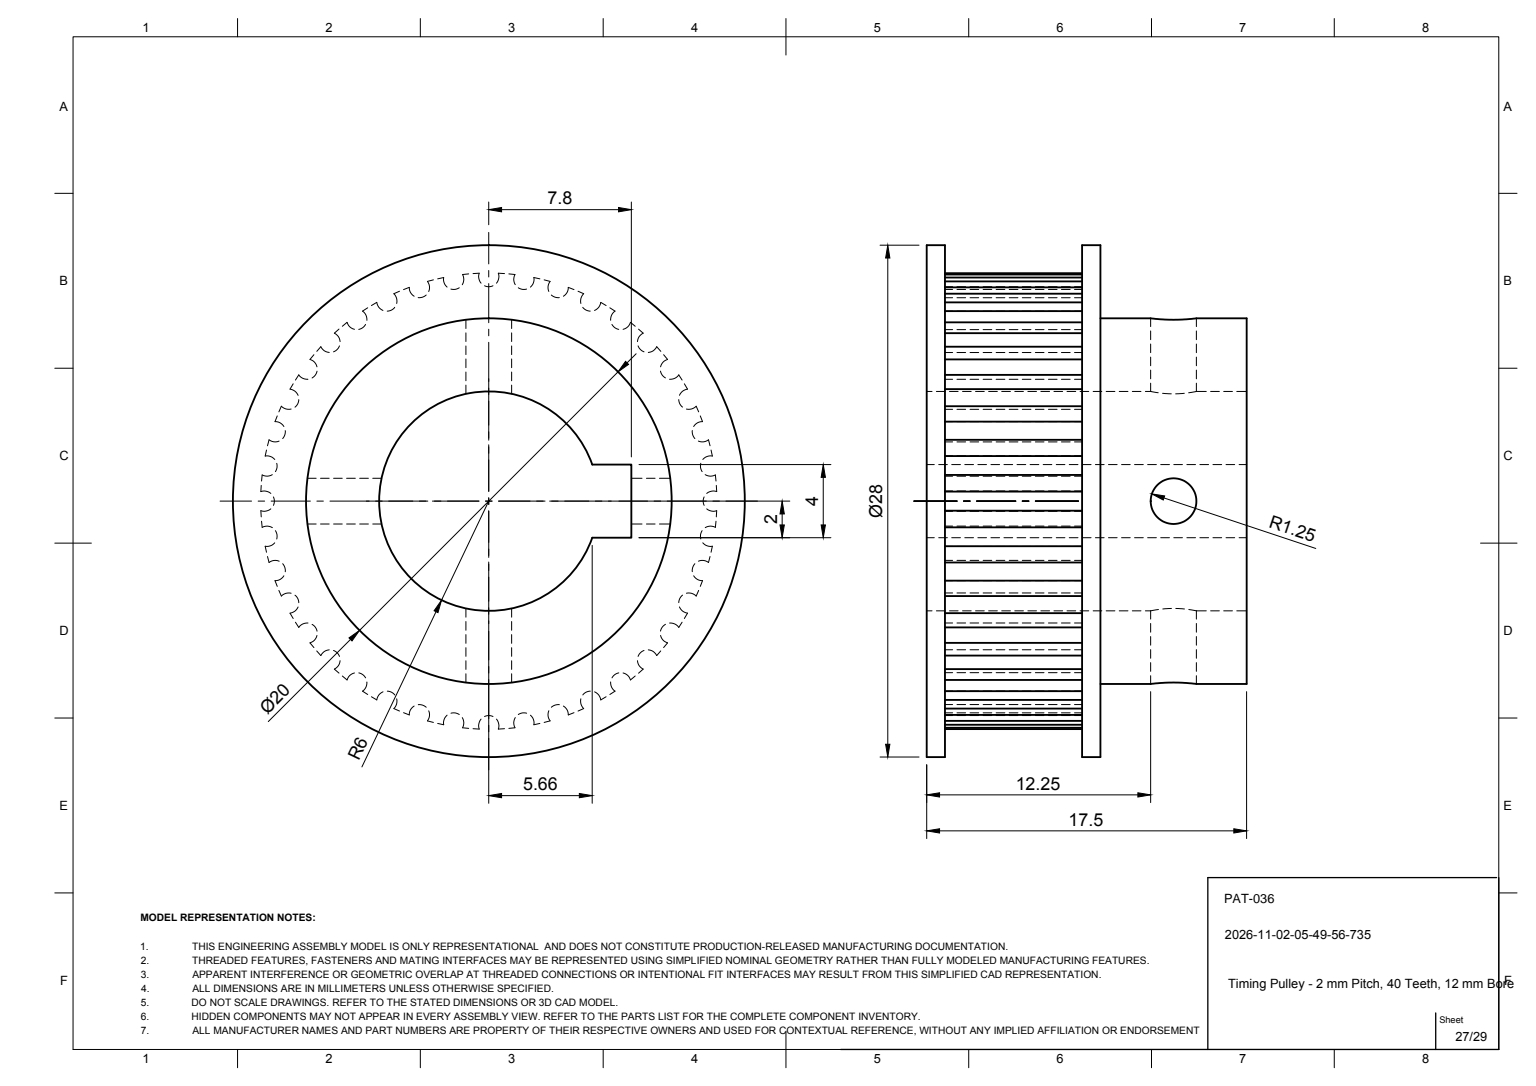
ISO-10303-21;
HEADER;
/* Generated by software containing ST-Developer
 * from STEP Tools, Inc. (www.steptools.com) 
 */

FILE_DESCRIPTION(
/* description */ ('Flange-mounted spindle'),
/* implementation_level */ '2;1');

FILE_NAME(
/* name */ 'Timing Pulley - 2 mm Pitch, 40 Teeth, 12 mm Bore.step',
/* time_stamp */ '2026-10-27T10:49:51-07:00',
/* author */ (''),
/* organization */ (''),
/* preprocessor_version */ 'ST-DEVELOPER v20.2',
/* originating_system */ 'Autodesk Translation Framework v15.17.0.0',
/* authorisation */ '');

FILE_SCHEMA (('AUTOMOTIVE_DESIGN { 1 0 10303 214 3 1 1 }'));
ENDSEC;

DATA;
#10=MECHANICAL_DESIGN_GEOMETRIC_PRESENTATION_REPRESENTATION('',(#359),#11764);
#243=B_SPLINE_CURVE_WITH_KNOTS('',3,(#10553,#10554,#10555,#10556,#10557,
#10558,#10559,#10560,#10561,#10562,#10563,#10564,#10565,#10566,#10567,#10568,
#10569,#10570),.UNSPECIFIED.,.F.,.F.,(4,2,2,2,2,2,2,2,4),(0.,0.0472365751919841,
0.0944731503839683,0.14170659898184,0.188940047579712,0.236173496177583,
0.283406944775455,0.330643519967439,0.377880095159423),.UNSPECIFIED.);
#244=B_SPLINE_CURVE_WITH_KNOTS('',3,(#10571,#10572,#10573,#10574,#10575,
#10576,#10577,#10578,#10579,#10580,#10581,#10582,#10583,#10584,#10585,#10586,
#10587,#10588),.UNSPECIFIED.,.F.,.F.,(4,2,2,2,2,2,2,2,4),(0.377880095159423,
0.425116670351408,0.472353245543392,0.519586694141263,0.566820142739135,
0.614053591337007,0.661287039934879,0.708523615126863,0.755760190318847),
 .UNSPECIFIED.);
#245=B_SPLINE_CURVE_WITH_KNOTS('',3,(#10591,#10592,#10593,#10594,#10595,
#10596,#10597,#10598,#10599,#10600,#10601,#10602,#10603,#10604,#10605,#10606,
#10607,#10608),.UNSPECIFIED.,.F.,.F.,(4,2,2,2,2,2,2,2,4),(0.,0.0472365751919841,
0.0944731503839682,0.14170659898184,0.188940047579712,0.236173496177583,
0.283406944775455,0.330643519967439,0.377880095159423),.UNSPECIFIED.);
#246=B_SPLINE_CURVE_WITH_KNOTS('',3,(#10609,#10610,#10611,#10612,#10613,
#10614,#10615,#10616,#10617,#10618,#10619,#10620,#10621,#10622,#10623,#10624,
#10625,#10626),.UNSPECIFIED.,.F.,.F.,(4,2,2,2,2,2,2,2,4),(0.377880095159423,
0.425116670351408,0.472353245543392,0.519586694141263,0.566820142739135,
0.614053591337007,0.661287039934879,0.708523615126863,0.755760190318847),
 .UNSPECIFIED.);
#247=B_SPLINE_CURVE_WITH_KNOTS('',3,(#10629,#10630,#10631,#10632,#10633,
#10634,#10635,#10636,#10637,#10638,#10639,#10640,#10641,#10642,#10643,#10644,
#10645,#10646),.UNSPECIFIED.,.F.,.F.,(4,2,2,2,2,2,2,2,4),(0.,0.0472365751919841,
0.0944731503839683,0.14170659898184,0.188940047579712,0.236173496177583,
0.283406944775455,0.330643519967439,0.377880095159423),.UNSPECIFIED.);
#248=B_SPLINE_CURVE_WITH_KNOTS('',3,(#10647,#10648,#10649,#10650,#10651,
#10652,#10653,#10654,#10655,#10656,#10657,#10658,#10659,#10660,#10661,#10662,
#10663,#10664),.UNSPECIFIED.,.F.,.F.,(4,2,2,2,2,2,2,2,4),(0.377880095159423,
0.425116670351408,0.472353245543392,0.519586694141263,0.566820142739135,
0.614053591337007,0.661287039934879,0.708523615126863,0.755760190318847),
 .UNSPECIFIED.);
#249=B_SPLINE_CURVE_WITH_KNOTS('',3,(#10668,#10669,#10670,#10671,#10672,
#10673,#10674,#10675,#10676,#10677),.UNSPECIFIED.,.F.,.F.,(4,2,2,2,4),(0.565665723963061,
0.61280433739166,0.659942950820258,0.70708195805217,0.754220965284082),
 .UNSPECIFIED.);
#250=B_SPLINE_CURVE_WITH_KNOTS('',3,(#10679,#10680,#10681,#10682,#10683,
#10684,#10685,#10686,#10687,#10688,#10689,#10690,#10691,#10692,#10693,#10694,
#10695,#10696),.UNSPECIFIED.,.F.,.F.,(4,2,2,2,2,2,2,2,4),(0.18855524132102,
0.235693854749619,0.282832468178217,0.329971475410129,0.377110482642041,
0.424249489873953,0.471388497105864,0.518527110534463,0.565665723963061),
 .UNSPECIFIED.);
#251=B_SPLINE_CURVE_WITH_KNOTS('',3,(#10697,#10698,#10699,#10700,#10701,
#10702,#10703,#10704,#10705,#10706),.UNSPECIFIED.,.F.,.F.,(4,2,2,2,4),(0.754220965284082,
0.801359972515993,0.848498979747905,0.895637593176504,0.942776206605102),
 .UNSPECIFIED.);
#252=B_SPLINE_CURVE_WITH_KNOTS('',3,(#10712,#10713,#10714,#10715,#10716,
#10717,#10718,#10719,#10720,#10721),.UNSPECIFIED.,.F.,.F.,(4,2,2,2,4),(0.565665723963061,
0.61280433739166,0.659942950820258,0.70708195805217,0.754220965284082),
 .UNSPECIFIED.);
#253=B_SPLINE_CURVE_WITH_KNOTS('',3,(#10723,#10724,#10725,#10726,#10727,
#10728,#10729,#10730,#10731,#10732,#10733,#10734,#10735,#10736,#10737,#10738,
#10739,#10740),.UNSPECIFIED.,.F.,.F.,(4,2,2,2,2,2,2,2,4),(0.18855524132102,
0.235693854749619,0.282832468178217,0.329971475410129,0.377110482642041,
0.424249489873953,0.471388497105864,0.518527110534463,0.565665723963061),
 .UNSPECIFIED.);
#254=B_SPLINE_CURVE_WITH_KNOTS('',3,(#10741,#10742,#10743,#10744,#10745,
#10746,#10747,#10748,#10749,#10750),.UNSPECIFIED.,.F.,.F.,(4,2,2,2,4),(0.754220965284082,
0.801359972515993,0.848498979747905,0.895637593176504,0.942776206605102),
 .UNSPECIFIED.);
#255=B_SPLINE_CURVE_WITH_KNOTS('',3,(#10760,#10761,#10762,#10763,#10764,
#10765,#10766,#10767,#10768,#10769,#10770,#10771,#10772,#10773,#10774,#10775,
#10776,#10777),.UNSPECIFIED.,.F.,.F.,(4,2,2,2,2,2,2,2,4),(0.18855524132102,
0.235693854749619,0.282832468178217,0.329971475410129,0.377110482642041,
0.424249489873953,0.471388497105864,0.518527110534463,0.565665723963061),
 .UNSPECIFIED.);
#256=B_SPLINE_CURVE_WITH_KNOTS('',3,(#10779,#10780,#10781,#10782,#10783,
#10784,#10785,#10786,#10787,#10788),.UNSPECIFIED.,.F.,.F.,(4,2,2,2,4),(0.565665723963061,
0.61280433739166,0.659942950820258,0.70708195805217,0.754220965284082),
 .UNSPECIFIED.);
#257=B_SPLINE_CURVE_WITH_KNOTS('',3,(#10789,#10790,#10791,#10792,#10793,
#10794,#10795,#10796,#10797,#10798),.UNSPECIFIED.,.F.,.F.,(4,2,2,2,4),(0.754220965284082,
0.801359972515993,0.848498979747905,0.895637593176504,0.942776206605102),
 .UNSPECIFIED.);
#258=B_SPLINE_CURVE_WITH_KNOTS('',3,(#10801,#10802,#10803,#10804,#10805,
#10806,#10807,#10808,#10809,#10810,#10811,#10812,#10813,#10814,#10815,#10816,
#10817,#10818),.UNSPECIFIED.,.F.,.F.,(4,2,2,2,2,2,2,2,4),(0.18855524132102,
0.235693854749619,0.282832468178217,0.329971475410129,0.377110482642041,
0.424249489873953,0.471388497105864,0.518527110534463,0.565665723963061),
 .UNSPECIFIED.);
#259=B_SPLINE_CURVE_WITH_KNOTS('',3,(#10820,#10821,#10822,#10823,#10824,
#10825,#10826,#10827,#10828,#10829),.UNSPECIFIED.,.F.,.F.,(4,2,2,2,4),(0.565665723963061,
0.61280433739166,0.659942950820258,0.70708195805217,0.754220965284082),
 .UNSPECIFIED.);
#260=B_SPLINE_CURVE_WITH_KNOTS('',3,(#10830,#10831,#10832,#10833,#10834,
#10835,#10836,#10837,#10838,#10839),.UNSPECIFIED.,.F.,.F.,(4,2,2,2,4),(0.754220965284082,
0.801359972515993,0.848498979747905,0.895637593176504,0.942776206605102),
 .UNSPECIFIED.);
#304=SHAPE_REPRESENTATION_RELATIONSHIP('SRR','None',#11902,#331);
#331=ADVANCED_BREP_SHAPE_REPRESENTATION('',(#385),#11757);
#359=STYLED_ITEM('',(#12092),#385);
#385=MANIFOLD_SOLID_BREP('Body1',#6153);
#488=FACE_BOUND('',#1303,.T.);
#489=FACE_BOUND('',#1306,.T.);
#490=FACE_BOUND('',#1308,.T.);
#491=FACE_BOUND('',#1309,.T.);
#492=FACE_BOUND('',#1310,.T.);
#493=FACE_BOUND('',#1314,.T.);
#494=FACE_BOUND('',#1315,.T.);
#495=FACE_BOUND('',#1316,.T.);
#496=FACE_BOUND('',#1320,.T.);
#497=FACE_BOUND('',#1322,.T.);
#498=FACE_BOUND('',#1325,.T.);
#499=FACE_BOUND('',#1327,.T.);
#616=PLANE('',#6808);
#617=PLANE('',#6809);
#618=PLANE('',#6811);
#619=PLANE('',#6812);
#620=PLANE('',#6824);
#621=PLANE('',#6825);
#622=PLANE('',#6909);
#623=PLANE('',#6910);
#859=FACE_OUTER_BOUND('',#1301,.T.);
#860=FACE_OUTER_BOUND('',#1302,.T.);
#861=FACE_OUTER_BOUND('',#1304,.T.);
#862=FACE_OUTER_BOUND('',#1305,.T.);
#863=FACE_OUTER_BOUND('',#1307,.T.);
#864=FACE_OUTER_BOUND('',#1311,.T.);
#865=FACE_OUTER_BOUND('',#1312,.T.);
#866=FACE_OUTER_BOUND('',#1313,.T.);
#867=FACE_OUTER_BOUND('',#1317,.T.);
#868=FACE_OUTER_BOUND('',#1318,.T.);
#869=FACE_OUTER_BOUND('',#1319,.T.);
#870=FACE_OUTER_BOUND('',#1321,.T.);
#871=FACE_OUTER_BOUND('',#1323,.T.);
#872=FACE_OUTER_BOUND('',#1324,.T.);
#873=FACE_OUTER_BOUND('',#1326,.T.);
#874=FACE_OUTER_BOUND('',#1328,.T.);
#875=FACE_OUTER_BOUND('',#1329,.T.);
#876=FACE_OUTER_BOUND('',#1330,.T.);
#877=FACE_OUTER_BOUND('',#1331,.T.);
#878=FACE_OUTER_BOUND('',#1332,.T.);
#879=FACE_OUTER_BOUND('',#1333,.T.);
#880=FACE_OUTER_BOUND('',#1334,.T.);
#881=FACE_OUTER_BOUND('',#1335,.T.);
#882=FACE_OUTER_BOUND('',#1336,.T.);
#883=FACE_OUTER_BOUND('',#1337,.T.);
#884=FACE_OUTER_BOUND('',#1338,.T.);
#885=FACE_OUTER_BOUND('',#1339,.T.);
#886=FACE_OUTER_BOUND('',#1340,.T.);
#887=FACE_OUTER_BOUND('',#1341,.T.);
#888=FACE_OUTER_BOUND('',#1342,.T.);
#889=FACE_OUTER_BOUND('',#1343,.T.);
#890=FACE_OUTER_BOUND('',#1344,.T.);
#891=FACE_OUTER_BOUND('',#1345,.T.);
#892=FACE_OUTER_BOUND('',#1346,.T.);
#893=FACE_OUTER_BOUND('',#1347,.T.);
#894=FACE_OUTER_BOUND('',#1348,.T.);
#895=FACE_OUTER_BOUND('',#1349,.T.);
#896=FACE_OUTER_BOUND('',#1350,.T.);
#897=FACE_OUTER_BOUND('',#1351,.T.);
#898=FACE_OUTER_BOUND('',#1352,.T.);
#899=FACE_OUTER_BOUND('',#1353,.T.);
#900=FACE_OUTER_BOUND('',#1354,.T.);
#901=FACE_OUTER_BOUND('',#1355,.T.);
#902=FACE_OUTER_BOUND('',#1356,.T.);
#903=FACE_OUTER_BOUND('',#1357,.T.);
#904=FACE_OUTER_BOUND('',#1358,.T.);
#905=FACE_OUTER_BOUND('',#1359,.T.);
#906=FACE_OUTER_BOUND('',#1360,.T.);
#907=FACE_OUTER_BOUND('',#1361,.T.);
#908=FACE_OUTER_BOUND('',#1362,.T.);
#909=FACE_OUTER_BOUND('',#1363,.T.);
#910=FACE_OUTER_BOUND('',#1364,.T.);
#911=FACE_OUTER_BOUND('',#1365,.T.);
#912=FACE_OUTER_BOUND('',#1366,.T.);
#913=FACE_OUTER_BOUND('',#1367,.T.);
#914=FACE_OUTER_BOUND('',#1368,.T.);
#915=FACE_OUTER_BOUND('',#1369,.T.);
#916=FACE_OUTER_BOUND('',#1370,.T.);
#917=FACE_OUTER_BOUND('',#1371,.T.);
#918=FACE_OUTER_BOUND('',#1372,.T.);
#919=FACE_OUTER_BOUND('',#1373,.T.);
#920=FACE_OUTER_BOUND('',#1374,.T.);
#921=FACE_OUTER_BOUND('',#1375,.T.);
#922=FACE_OUTER_BOUND('',#1376,.T.);
#923=FACE_OUTER_BOUND('',#1377,.T.);
#924=FACE_OUTER_BOUND('',#1378,.T.);
#925=FACE_OUTER_BOUND('',#1379,.T.);
#926=FACE_OUTER_BOUND('',#1380,.T.);
#927=FACE_OUTER_BOUND('',#1381,.T.);
#928=FACE_OUTER_BOUND('',#1382,.T.);
#929=FACE_OUTER_BOUND('',#1383,.T.);
#930=FACE_OUTER_BOUND('',#1384,.T.);
#931=FACE_OUTER_BOUND('',#1385,.T.);
#932=FACE_OUTER_BOUND('',#1386,.T.);
#933=FACE_OUTER_BOUND('',#1387,.T.);
#934=FACE_OUTER_BOUND('',#1388,.T.);
#935=FACE_OUTER_BOUND('',#1389,.T.);
#936=FACE_OUTER_BOUND('',#1390,.T.);
#937=FACE_OUTER_BOUND('',#1391,.T.);
#938=FACE_OUTER_BOUND('',#1392,.T.);
#939=FACE_OUTER_BOUND('',#1393,.T.);
#940=FACE_OUTER_BOUND('',#1394,.T.);
#941=FACE_OUTER_BOUND('',#1395,.T.);
#942=FACE_OUTER_BOUND('',#1396,.T.);
#943=FACE_OUTER_BOUND('',#1397,.T.);
#944=FACE_OUTER_BOUND('',#1398,.T.);
#945=FACE_OUTER_BOUND('',#1399,.T.);
#946=FACE_OUTER_BOUND('',#1400,.T.);
#947=FACE_OUTER_BOUND('',#1401,.T.);
#948=FACE_OUTER_BOUND('',#1402,.T.);
#949=FACE_OUTER_BOUND('',#1403,.T.);
#950=FACE_OUTER_BOUND('',#1404,.T.);
#951=FACE_OUTER_BOUND('',#1405,.T.);
#952=FACE_OUTER_BOUND('',#1406,.T.);
#953=FACE_OUTER_BOUND('',#1407,.T.);
#954=FACE_OUTER_BOUND('',#1408,.T.);
#1301=EDGE_LOOP('',(#4783,#4784,#4785,#4786));
#1302=EDGE_LOOP('',(#4787,#4788,#4789,#4790));
#1303=EDGE_LOOP('',(#4791));
#1304=EDGE_LOOP('',(#4792,#4793,#4794,#4795));
#1305=EDGE_LOOP('',(#4796));
#1306=EDGE_LOOP('',(#4797,#4798,#4799,#4800));
#1307=EDGE_LOOP('',(#4801,#4802,#4803,#4804));
#1308=EDGE_LOOP('',(#4805,#4806));
#1309=EDGE_LOOP('',(#4807,#4808));
#1310=EDGE_LOOP('',(#4809,#4810));
#1311=EDGE_LOOP('',(#4811,#4812,#4813,#4814,#4815,#4816,#4817));
#1312=EDGE_LOOP('',(#4818,#4819,#4820,#4821,#4822,#4823,#4824));
#1313=EDGE_LOOP('',(#4825,#4826,#4827,#4828,#4829,#4830,#4831,#4832,#4833));
#1314=EDGE_LOOP('',(#4834,#4835,#4836));
#1315=EDGE_LOOP('',(#4837,#4838,#4839));
#1316=EDGE_LOOP('',(#4840,#4841,#4842));
#1317=EDGE_LOOP('',(#4843,#4844,#4845,#4846,#4847,#4848));
#1318=EDGE_LOOP('',(#4849,#4850,#4851,#4852,#4853,#4854,#4855));
#1319=EDGE_LOOP('',(#4856));
#1320=EDGE_LOOP('',(#4857,#4858,#4859,#4860));
#1321=EDGE_LOOP('',(#4861));
#1322=EDGE_LOOP('',(#4862,#4863,#4864,#4865,#4866,#4867,#4868,#4869,#4870,
#4871,#4872,#4873,#4874,#4875,#4876,#4877,#4878,#4879,#4880,#4881,#4882,
#4883,#4884,#4885,#4886,#4887,#4888,#4889,#4890,#4891,#4892,#4893,#4894,
#4895,#4896,#4897,#4898,#4899,#4900,#4901,#4902,#4903,#4904,#4905,#4906,
#4907,#4908,#4909,#4910,#4911,#4912,#4913,#4914,#4915,#4916,#4917,#4918,
#4919,#4920,#4921,#4922,#4923,#4924,#4925,#4926,#4927,#4928,#4929,#4930,
#4931,#4932,#4933,#4934,#4935,#4936,#4937,#4938,#4939,#4940,#4941));
#1323=EDGE_LOOP('',(#4942,#4943,#4944,#4945));
#1324=EDGE_LOOP('',(#4946));
#1325=EDGE_LOOP('',(#4947));
#1326=EDGE_LOOP('',(#4948));
#1327=EDGE_LOOP('',(#4949,#4950,#4951,#4952,#4953,#4954,#4955,#4956,#4957,
#4958,#4959,#4960,#4961,#4962,#4963,#4964,#4965,#4966,#4967,#4968,#4969,
#4970,#4971,#4972,#4973,#4974,#4975,#4976,#4977,#4978,#4979,#4980,#4981,
#4982,#4983,#4984,#4985,#4986,#4987,#4988,#4989,#4990,#4991,#4992,#4993,
#4994,#4995,#4996,#4997,#4998,#4999,#5000,#5001,#5002,#5003,#5004,#5005,
#5006,#5007,#5008,#5009,#5010,#5011,#5012,#5013,#5014,#5015,#5016,#5017,
#5018,#5019,#5020,#5021,#5022,#5023,#5024,#5025,#5026,#5027,#5028));
#1328=EDGE_LOOP('',(#5029,#5030,#5031,#5032));
#1329=EDGE_LOOP('',(#5033,#5034,#5035,#5036));
#1330=EDGE_LOOP('',(#5037,#5038,#5039,#5040));
#1331=EDGE_LOOP('',(#5041,#5042,#5043,#5044));
#1332=EDGE_LOOP('',(#5045,#5046,#5047,#5048));
#1333=EDGE_LOOP('',(#5049,#5050,#5051,#5052));
#1334=EDGE_LOOP('',(#5053,#5054,#5055,#5056));
#1335=EDGE_LOOP('',(#5057,#5058,#5059,#5060));
#1336=EDGE_LOOP('',(#5061,#5062,#5063,#5064));
#1337=EDGE_LOOP('',(#5065,#5066,#5067,#5068));
#1338=EDGE_LOOP('',(#5069,#5070,#5071,#5072));
#1339=EDGE_LOOP('',(#5073,#5074,#5075,#5076));
#1340=EDGE_LOOP('',(#5077,#5078,#5079,#5080));
#1341=EDGE_LOOP('',(#5081,#5082,#5083,#5084));
#1342=EDGE_LOOP('',(#5085,#5086,#5087,#5088));
#1343=EDGE_LOOP('',(#5089,#5090,#5091,#5092));
#1344=EDGE_LOOP('',(#5093,#5094,#5095,#5096));
#1345=EDGE_LOOP('',(#5097,#5098,#5099,#5100));
#1346=EDGE_LOOP('',(#5101,#5102,#5103,#5104));
#1347=EDGE_LOOP('',(#5105,#5106,#5107,#5108));
#1348=EDGE_LOOP('',(#5109,#5110,#5111,#5112));
#1349=EDGE_LOOP('',(#5113,#5114,#5115,#5116));
#1350=EDGE_LOOP('',(#5117,#5118,#5119,#5120));
#1351=EDGE_LOOP('',(#5121,#5122,#5123,#5124));
#1352=EDGE_LOOP('',(#5125,#5126,#5127,#5128));
#1353=EDGE_LOOP('',(#5129,#5130,#5131,#5132));
#1354=EDGE_LOOP('',(#5133,#5134,#5135,#5136));
#1355=EDGE_LOOP('',(#5137,#5138,#5139,#5140));
#1356=EDGE_LOOP('',(#5141,#5142,#5143,#5144));
#1357=EDGE_LOOP('',(#5145,#5146,#5147,#5148));
#1358=EDGE_LOOP('',(#5149,#5150,#5151,#5152));
#1359=EDGE_LOOP('',(#5153,#5154,#5155,#5156));
#1360=EDGE_LOOP('',(#5157,#5158,#5159,#5160));
#1361=EDGE_LOOP('',(#5161,#5162,#5163,#5164));
#1362=EDGE_LOOP('',(#5165,#5166,#5167,#5168));
#1363=EDGE_LOOP('',(#5169,#5170,#5171,#5172));
#1364=EDGE_LOOP('',(#5173,#5174,#5175,#5176));
#1365=EDGE_LOOP('',(#5177,#5178,#5179,#5180));
#1366=EDGE_LOOP('',(#5181,#5182,#5183,#5184));
#1367=EDGE_LOOP('',(#5185,#5186,#5187,#5188));
#1368=EDGE_LOOP('',(#5189,#5190,#5191,#5192));
#1369=EDGE_LOOP('',(#5193,#5194,#5195,#5196));
#1370=EDGE_LOOP('',(#5197,#5198,#5199,#5200));
#1371=EDGE_LOOP('',(#5201,#5202,#5203,#5204));
#1372=EDGE_LOOP('',(#5205,#5206,#5207,#5208));
#1373=EDGE_LOOP('',(#5209,#5210,#5211,#5212));
#1374=EDGE_LOOP('',(#5213,#5214,#5215,#5216));
#1375=EDGE_LOOP('',(#5217,#5218,#5219,#5220));
#1376=EDGE_LOOP('',(#5221,#5222,#5223,#5224));
#1377=EDGE_LOOP('',(#5225,#5226,#5227,#5228));
#1378=EDGE_LOOP('',(#5229,#5230,#5231,#5232));
#1379=EDGE_LOOP('',(#5233,#5234,#5235,#5236));
#1380=EDGE_LOOP('',(#5237,#5238,#5239,#5240));
#1381=EDGE_LOOP('',(#5241,#5242,#5243,#5244));
#1382=EDGE_LOOP('',(#5245,#5246,#5247,#5248));
#1383=EDGE_LOOP('',(#5249,#5250,#5251,#5252));
#1384=EDGE_LOOP('',(#5253,#5254,#5255,#5256));
#1385=EDGE_LOOP('',(#5257,#5258,#5259,#5260));
#1386=EDGE_LOOP('',(#5261,#5262,#5263,#5264));
#1387=EDGE_LOOP('',(#5265,#5266,#5267,#5268));
#1388=EDGE_LOOP('',(#5269,#5270,#5271,#5272));
#1389=EDGE_LOOP('',(#5273,#5274,#5275,#5276));
#1390=EDGE_LOOP('',(#5277,#5278,#5279,#5280));
#1391=EDGE_LOOP('',(#5281,#5282,#5283,#5284));
#1392=EDGE_LOOP('',(#5285,#5286,#5287,#5288));
#1393=EDGE_LOOP('',(#5289,#5290,#5291,#5292));
#1394=EDGE_LOOP('',(#5293,#5294,#5295,#5296));
#1395=EDGE_LOOP('',(#5297,#5298,#5299,#5300));
#1396=EDGE_LOOP('',(#5301,#5302,#5303,#5304));
#1397=EDGE_LOOP('',(#5305,#5306,#5307,#5308));
#1398=EDGE_LOOP('',(#5309,#5310,#5311,#5312));
#1399=EDGE_LOOP('',(#5313,#5314,#5315,#5316));
#1400=EDGE_LOOP('',(#5317,#5318,#5319,#5320));
#1401=EDGE_LOOP('',(#5321,#5322,#5323,#5324));
#1402=EDGE_LOOP('',(#5325,#5326,#5327,#5328));
#1403=EDGE_LOOP('',(#5329,#5330,#5331,#5332));
#1404=EDGE_LOOP('',(#5333,#5334,#5335,#5336));
#1405=EDGE_LOOP('',(#5337,#5338,#5339,#5340));
#1406=EDGE_LOOP('',(#5341,#5342,#5343,#5344));
#1407=EDGE_LOOP('',(#5345,#5346,#5347,#5348));
#1408=EDGE_LOOP('',(#5349,#5350,#5351,#5352));
#1699=LINE('',#10525,#2121);
#1700=LINE('',#10527,#2122);
#1701=LINE('',#10529,#2123);
#1702=LINE('',#10530,#2124);
#1703=LINE('',#10533,#2125);
#1704=LINE('',#10535,#2126);
#1705=LINE('',#10536,#2127);
#1706=LINE('',#10541,#2128);
#1707=LINE('',#10543,#2129);
#1708=LINE('',#10544,#2130);
#1709=LINE('',#10707,#2131);
#1710=LINE('',#10710,#2132);
#1711=LINE('',#10754,#2133);
#1712=LINE('',#10756,#2134);
#1713=LINE('',#10841,#2135);
#1714=LINE('',#10843,#2136);
#1715=LINE('',#11011,#2137);
#1716=LINE('',#11177,#2138);
#1717=LINE('',#11179,#2139);
#1718=LINE('',#11180,#2140);
#1719=LINE('',#11182,#2141);
#1720=LINE('',#11184,#2142);
#1721=LINE('',#11186,#2143);
#1722=LINE('',#11188,#2144);
#1723=LINE('',#11190,#2145);
#1724=LINE('',#11192,#2146);
#1725=LINE('',#11194,#2147);
#1726=LINE('',#11196,#2148);
#1727=LINE('',#11198,#2149);
#1728=LINE('',#11200,#2150);
#1729=LINE('',#11202,#2151);
#1730=LINE('',#11204,#2152);
#1731=LINE('',#11206,#2153);
#1732=LINE('',#11208,#2154);
#1733=LINE('',#11210,#2155);
#1734=LINE('',#11212,#2156);
#1735=LINE('',#11214,#2157);
#1736=LINE('',#11216,#2158);
#1737=LINE('',#11218,#2159);
#1738=LINE('',#11220,#2160);
#1739=LINE('',#11222,#2161);
#1740=LINE('',#11224,#2162);
#1741=LINE('',#11226,#2163);
#1742=LINE('',#11228,#2164);
#1743=LINE('',#11230,#2165);
#1744=LINE('',#11232,#2166);
#1745=LINE('',#11234,#2167);
#1746=LINE('',#11236,#2168);
#1747=LINE('',#11238,#2169);
#1748=LINE('',#11240,#2170);
#1749=LINE('',#11242,#2171);
#1750=LINE('',#11244,#2172);
#1751=LINE('',#11246,#2173);
#1752=LINE('',#11248,#2174);
#1753=LINE('',#11250,#2175);
#1754=LINE('',#11252,#2176);
#1755=LINE('',#11254,#2177);
#1756=LINE('',#11256,#2178);
#1757=LINE('',#11258,#2179);
#1758=LINE('',#11260,#2180);
#1759=LINE('',#11262,#2181);
#1760=LINE('',#11264,#2182);
#1761=LINE('',#11266,#2183);
#1762=LINE('',#11268,#2184);
#1763=LINE('',#11270,#2185);
#1764=LINE('',#11272,#2186);
#1765=LINE('',#11274,#2187);
#1766=LINE('',#11276,#2188);
#1767=LINE('',#11278,#2189);
#1768=LINE('',#11280,#2190);
#1769=LINE('',#11282,#2191);
#1770=LINE('',#11284,#2192);
#1771=LINE('',#11286,#2193);
#1772=LINE('',#11288,#2194);
#1773=LINE('',#11290,#2195);
#1774=LINE('',#11292,#2196);
#1775=LINE('',#11294,#2197);
#1776=LINE('',#11296,#2198);
#1777=LINE('',#11298,#2199);
#1778=LINE('',#11300,#2200);
#1779=LINE('',#11302,#2201);
#1780=LINE('',#11304,#2202);
#1781=LINE('',#11306,#2203);
#1782=LINE('',#11308,#2204);
#1783=LINE('',#11310,#2205);
#1784=LINE('',#11312,#2206);
#1785=LINE('',#11314,#2207);
#1786=LINE('',#11316,#2208);
#1787=LINE('',#11318,#2209);
#1788=LINE('',#11320,#2210);
#1789=LINE('',#11322,#2211);
#1790=LINE('',#11324,#2212);
#1791=LINE('',#11326,#2213);
#1792=LINE('',#11328,#2214);
#1793=LINE('',#11330,#2215);
#1794=LINE('',#11332,#2216);
#1795=LINE('',#11334,#2217);
#1796=LINE('',#11336,#2218);
#2121=VECTOR('',#8128,1.);
#2122=VECTOR('',#8129,1.);
#2123=VECTOR('',#8130,1.);
#2124=VECTOR('',#8131,1.);
#2125=VECTOR('',#8134,1.);
#2126=VECTOR('',#8135,1.);
#2127=VECTOR('',#8136,1.);
#2128=VECTOR('',#8141,1.);
#2129=VECTOR('',#8142,1.);
#2130=VECTOR('',#8143,1.);
#2131=VECTOR('',#8156,0.125);
#2132=VECTOR('',#8159,0.125);
#2133=VECTOR('',#8164,1.);
#2134=VECTOR('',#8165,1.);
#2135=VECTOR('',#8170,0.125);
#2136=VECTOR('',#8173,0.125);
#2137=VECTOR('',#8344,1.4);
#2138=VECTOR('',#8513,1.4);
#2139=VECTOR('',#8516,1.);
#2140=VECTOR('',#8517,1.);
#2141=VECTOR('',#8520,1.);
#2142=VECTOR('',#8523,1.);
#2143=VECTOR('',#8526,1.);
#2144=VECTOR('',#8529,1.);
#2145=VECTOR('',#8532,1.);
#2146=VECTOR('',#8535,1.);
#2147=VECTOR('',#8538,1.);
#2148=VECTOR('',#8541,1.);
#2149=VECTOR('',#8544,1.);
#2150=VECTOR('',#8547,1.);
#2151=VECTOR('',#8550,1.);
#2152=VECTOR('',#8553,1.);
#2153=VECTOR('',#8556,1.);
#2154=VECTOR('',#8559,1.);
#2155=VECTOR('',#8562,1.);
#2156=VECTOR('',#8565,1.);
#2157=VECTOR('',#8568,1.);
#2158=VECTOR('',#8571,1.);
#2159=VECTOR('',#8574,1.);
#2160=VECTOR('',#8577,1.);
#2161=VECTOR('',#8580,1.);
#2162=VECTOR('',#8583,1.);
#2163=VECTOR('',#8586,1.);
#2164=VECTOR('',#8589,1.);
#2165=VECTOR('',#8592,1.);
#2166=VECTOR('',#8595,1.);
#2167=VECTOR('',#8598,1.);
#2168=VECTOR('',#8601,1.);
#2169=VECTOR('',#8604,1.);
#2170=VECTOR('',#8607,1.);
#2171=VECTOR('',#8610,1.);
#2172=VECTOR('',#8613,1.);
#2173=VECTOR('',#8616,1.);
#2174=VECTOR('',#8619,1.);
#2175=VECTOR('',#8622,1.);
#2176=VECTOR('',#8625,1.);
#2177=VECTOR('',#8628,1.);
#2178=VECTOR('',#8631,1.);
#2179=VECTOR('',#8634,1.);
#2180=VECTOR('',#8637,1.);
#2181=VECTOR('',#8640,1.);
#2182=VECTOR('',#8643,1.);
#2183=VECTOR('',#8646,1.);
#2184=VECTOR('',#8649,1.);
#2185=VECTOR('',#8652,1.);
#2186=VECTOR('',#8655,1.);
#2187=VECTOR('',#8658,1.);
#2188=VECTOR('',#8661,1.);
#2189=VECTOR('',#8664,1.);
#2190=VECTOR('',#8667,1.);
#2191=VECTOR('',#8670,1.);
#2192=VECTOR('',#8673,1.);
#2193=VECTOR('',#8676,1.);
#2194=VECTOR('',#8679,1.);
#2195=VECTOR('',#8682,1.);
#2196=VECTOR('',#8685,1.);
#2197=VECTOR('',#8688,1.);
#2198=VECTOR('',#8691,1.);
#2199=VECTOR('',#8694,1.);
#2200=VECTOR('',#8697,1.);
#2201=VECTOR('',#8700,1.);
#2202=VECTOR('',#8703,1.);
#2203=VECTOR('',#8706,1.);
#2204=VECTOR('',#8709,1.);
#2205=VECTOR('',#8712,1.);
#2206=VECTOR('',#8715,1.);
#2207=VECTOR('',#8718,1.);
#2208=VECTOR('',#8721,1.);
#2209=VECTOR('',#8724,1.);
#2210=VECTOR('',#8727,1.);
#2211=VECTOR('',#8730,1.);
#2212=VECTOR('',#8733,1.);
#2213=VECTOR('',#8736,1.);
#2214=VECTOR('',#8739,1.);
#2215=VECTOR('',#8742,1.);
#2216=VECTOR('',#8745,1.);
#2217=VECTOR('',#8748,1.);
#2218=VECTOR('',#8751,1.);
#2460=CIRCLE('',#6810,0.125);
#2461=CIRCLE('',#6813,1.4);
#2462=CIRCLE('',#6814,0.6);
#2463=CIRCLE('',#6816,0.6);
#2464=CIRCLE('',#6820,1.);
#2465=CIRCLE('',#6821,1.);
#2466=CIRCLE('',#6826,1.4);
#2467=CIRCLE('',#6827,0.0555000000000001);
#2468=CIRCLE('',#6828,1.24783954473516);
#2469=CIRCLE('',#6829,0.0555000000000001);
#2470=CIRCLE('',#6830,1.24783954473516);
#2471=CIRCLE('',#6831,0.0555000000000001);
#2472=CIRCLE('',#6832,1.24783954473516);
#2473=CIRCLE('',#6833,0.0555000000000001);
#2474=CIRCLE('',#6834,1.24783954473516);
#2475=CIRCLE('',#6835,0.0555000000000001);
#2476=CIRCLE('',#6836,1.24783954473516);
#2477=CIRCLE('',#6837,0.0555000000000001);
#2478=CIRCLE('',#6838,1.24783954473516);
#2479=CIRCLE('',#6839,0.0555000000000001);
#2480=CIRCLE('',#6840,1.24783954473516);
#2481=CIRCLE('',#6841,0.0555000000000001);
#2482=CIRCLE('',#6842,1.24783954473516);
#2483=CIRCLE('',#6843,0.0555000000000001);
#2484=CIRCLE('',#6844,1.24783954473516);
#2485=CIRCLE('',#6845,0.0555000000000001);
#2486=CIRCLE('',#6846,1.24783954473516);
#2487=CIRCLE('',#6847,0.0555000000000001);
#2488=CIRCLE('',#6848,1.24783954473516);
#2489=CIRCLE('',#6849,0.0555000000000001);
#2490=CIRCLE('',#6850,1.24783954473516);
#2491=CIRCLE('',#6851,0.0555000000000001);
#2492=CIRCLE('',#6852,1.24783954473516);
#2493=CIRCLE('',#6853,0.0555000000000001);
#2494=CIRCLE('',#6854,1.24783954473516);
#2495=CIRCLE('',#6855,0.0555000000000001);
#2496=CIRCLE('',#6856,1.24783954473516);
#2497=CIRCLE('',#6857,0.0555000000000001);
#2498=CIRCLE('',#6858,1.24783954473516);
#2499=CIRCLE('',#6859,0.0555000000000001);
#2500=CIRCLE('',#6860,1.24783954473516);
#2501=CIRCLE('',#6861,0.0555000000000001);
#2502=CIRCLE('',#6862,1.24783954473516);
#2503=CIRCLE('',#6863,0.0555000000000001);
#2504=CIRCLE('',#6864,1.24783954473516);
#2505=CIRCLE('',#6865,0.0555000000000001);
#2506=CIRCLE('',#6866,1.24783954473516);
#2507=CIRCLE('',#6867,0.0555000000000001);
#2508=CIRCLE('',#6868,1.24783954473516);
#2509=CIRCLE('',#6869,0.0555000000000001);
#2510=CIRCLE('',#6870,1.24783954473516);
#2511=CIRCLE('',#6871,0.0555000000000001);
#2512=CIRCLE('',#6872,1.24783954473516);
#2513=CIRCLE('',#6873,0.0555000000000001);
#2514=CIRCLE('',#6874,1.24783954473516);
#2515=CIRCLE('',#6875,0.0555000000000001);
#2516=CIRCLE('',#6876,1.24783954473516);
#2517=CIRCLE('',#6877,0.0555000000000001);
#2518=CIRCLE('',#6878,1.24783954473516);
#2519=CIRCLE('',#6879,0.0555000000000001);
#2520=CIRCLE('',#6880,1.24783954473516);
#2521=CIRCLE('',#6881,0.0555000000000001);
#2522=CIRCLE('',#6882,1.24783954473516);
#2523=CIRCLE('',#6883,0.0555000000000001);
#2524=CIRCLE('',#6884,1.24783954473516);
#2525=CIRCLE('',#6885,0.0555000000000001);
#2526=CIRCLE('',#6886,1.24783954473516);
#2527=CIRCLE('',#6887,0.0555000000000001);
#2528=CIRCLE('',#6888,1.24783954473516);
#2529=CIRCLE('',#6889,0.0555000000000001);
#2530=CIRCLE('',#6890,1.24783954473516);
#2531=CIRCLE('',#6891,0.0555000000000001);
#2532=CIRCLE('',#6892,1.24783954473516);
#2533=CIRCLE('',#6893,0.0555000000000001);
#2534=CIRCLE('',#6894,1.24783954473516);
#2535=CIRCLE('',#6895,0.0555000000000001);
#2536=CIRCLE('',#6896,1.24783954473516);
#2537=CIRCLE('',#6897,0.0555000000000001);
#2538=CIRCLE('',#6898,1.24783954473516);
#2539=CIRCLE('',#6899,0.0555000000000001);
#2540=CIRCLE('',#6900,1.24783954473516);
#2541=CIRCLE('',#6901,0.0555000000000001);
#2542=CIRCLE('',#6902,1.24783954473516);
#2543=CIRCLE('',#6903,0.0555000000000001);
#2544=CIRCLE('',#6904,1.24783954473516);
#2545=CIRCLE('',#6905,0.0555000000000001);
#2546=CIRCLE('',#6906,1.24783954473516);
#2547=CIRCLE('',#6908,1.4);
#2548=CIRCLE('',#6911,1.4);
#2549=CIRCLE('',#6912,0.0555000000000001);
#2550=CIRCLE('',#6913,1.24783954473516);
#2551=CIRCLE('',#6914,0.0555000000000001);
#2552=CIRCLE('',#6915,1.24783954473516);
#2553=CIRCLE('',#6916,0.0555000000000001);
#2554=CIRCLE('',#6917,1.24783954473516);
#2555=CIRCLE('',#6918,0.0555000000000001);
#2556=CIRCLE('',#6919,1.24783954473516);
#2557=CIRCLE('',#6920,0.0555000000000001);
#2558=CIRCLE('',#6921,1.24783954473516);
#2559=CIRCLE('',#6922,0.0555000000000001);
#2560=CIRCLE('',#6923,1.24783954473516);
#2561=CIRCLE('',#6924,0.0555000000000001);
#2562=CIRCLE('',#6925,1.24783954473516);
#2563=CIRCLE('',#6926,0.0555000000000001);
#2564=CIRCLE('',#6927,1.24783954473516);
#2565=CIRCLE('',#6928,0.0555000000000001);
#2566=CIRCLE('',#6929,1.24783954473516);
#2567=CIRCLE('',#6930,0.0555000000000001);
#2568=CIRCLE('',#6931,1.24783954473516);
#2569=CIRCLE('',#6932,0.0555000000000001);
#2570=CIRCLE('',#6933,1.24783954473516);
#2571=CIRCLE('',#6934,0.0555000000000001);
#2572=CIRCLE('',#6935,1.24783954473516);
#2573=CIRCLE('',#6936,0.0555000000000001);
#2574=CIRCLE('',#6937,1.24783954473516);
#2575=CIRCLE('',#6938,0.0555000000000001);
#2576=CIRCLE('',#6939,1.24783954473516);
#2577=CIRCLE('',#6940,0.0555000000000001);
#2578=CIRCLE('',#6941,1.24783954473516);
#2579=CIRCLE('',#6942,0.0555000000000001);
#2580=CIRCLE('',#6943,1.24783954473516);
#2581=CIRCLE('',#6944,0.0555000000000001);
#2582=CIRCLE('',#6945,1.24783954473516);
#2583=CIRCLE('',#6946,0.0555000000000001);
#2584=CIRCLE('',#6947,1.24783954473516);
#2585=CIRCLE('',#6948,0.0555000000000001);
#2586=CIRCLE('',#6949,1.24783954473516);
#2587=CIRCLE('',#6950,0.0555000000000001);
#2588=CIRCLE('',#6951,1.24783954473516);
#2589=CIRCLE('',#6952,0.0555000000000001);
#2590=CIRCLE('',#6953,1.24783954473516);
#2591=CIRCLE('',#6954,0.0555000000000001);
#2592=CIRCLE('',#6955,1.24783954473516);
#2593=CIRCLE('',#6956,0.0555000000000001);
#2594=CIRCLE('',#6957,1.24783954473516);
#2595=CIRCLE('',#6958,0.0555000000000001);
#2596=CIRCLE('',#6959,1.24783954473516);
#2597=CIRCLE('',#6960,0.0555000000000001);
#2598=CIRCLE('',#6961,1.24783954473516);
#2599=CIRCLE('',#6962,0.0555000000000001);
#2600=CIRCLE('',#6963,1.24783954473516);
#2601=CIRCLE('',#6964,0.0555000000000001);
#2602=CIRCLE('',#6965,1.24783954473516);
#2603=CIRCLE('',#6966,0.0555000000000001);
#2604=CIRCLE('',#6967,1.24783954473516);
#2605=CIRCLE('',#6968,0.0555000000000001);
#2606=CIRCLE('',#6969,1.24783954473516);
#2607=CIRCLE('',#6970,0.0555000000000001);
#2608=CIRCLE('',#6971,1.24783954473516);
#2609=CIRCLE('',#6972,0.0555000000000001);
#2610=CIRCLE('',#6973,1.24783954473516);
#2611=CIRCLE('',#6974,0.0555000000000001);
#2612=CIRCLE('',#6975,1.24783954473516);
#2613=CIRCLE('',#6976,0.0555000000000001);
#2614=CIRCLE('',#6977,1.24783954473516);
#2615=CIRCLE('',#6978,0.0555000000000001);
#2616=CIRCLE('',#6979,1.24783954473516);
#2617=CIRCLE('',#6980,0.0555000000000001);
#2618=CIRCLE('',#6981,1.24783954473516);
#2619=CIRCLE('',#6982,0.0555000000000001);
#2620=CIRCLE('',#6983,1.24783954473516);
#2621=CIRCLE('',#6984,0.0555000000000001);
#2622=CIRCLE('',#6985,1.24783954473516);
#2623=CIRCLE('',#6986,0.0555000000000001);
#2624=CIRCLE('',#6987,1.24783954473516);
#2625=CIRCLE('',#6988,0.0555000000000001);
#2626=CIRCLE('',#6989,1.24783954473516);
#2627=CIRCLE('',#6990,0.0555000000000001);
#2628=CIRCLE('',#6991,1.24783954473516);
#2914=VERTEX_POINT('',#10523);
#2915=VERTEX_POINT('',#10524);
#2916=VERTEX_POINT('',#10526);
#2917=VERTEX_POINT('',#10528);
#2918=VERTEX_POINT('',#10532);
#2919=VERTEX_POINT('',#10534);
#2920=VERTEX_POINT('',#10537);
#2921=VERTEX_POINT('',#10540);
#2922=VERTEX_POINT('',#10542);
#2923=VERTEX_POINT('',#10546);
#2924=VERTEX_POINT('',#10551);
#2925=VERTEX_POINT('',#10552);
#2926=VERTEX_POINT('',#10589);
#2927=VERTEX_POINT('',#10590);
#2928=VERTEX_POINT('',#10627);
#2929=VERTEX_POINT('',#10628);
#2930=VERTEX_POINT('',#10666);
#2931=VERTEX_POINT('',#10667);
#2932=VERTEX_POINT('',#10678);
#2933=VERTEX_POINT('',#10709);
#2934=VERTEX_POINT('',#10711);
#2935=VERTEX_POINT('',#10722);
#2936=VERTEX_POINT('',#10752);
#2937=VERTEX_POINT('',#10755);
#2938=VERTEX_POINT('',#10758);
#2939=VERTEX_POINT('',#10759);
#2940=VERTEX_POINT('',#10778);
#2941=VERTEX_POINT('',#10799);
#2942=VERTEX_POINT('',#10800);
#2943=VERTEX_POINT('',#10819);
#2944=VERTEX_POINT('',#10846);
#2945=VERTEX_POINT('',#10848);
#2946=VERTEX_POINT('',#10849);
#2947=VERTEX_POINT('',#10851);
#2948=VERTEX_POINT('',#10853);
#2949=VERTEX_POINT('',#10855);
#2950=VERTEX_POINT('',#10857);
#2951=VERTEX_POINT('',#10859);
#2952=VERTEX_POINT('',#10861);
#2953=VERTEX_POINT('',#10863);
#2954=VERTEX_POINT('',#10865);
#2955=VERTEX_POINT('',#10867);
#2956=VERTEX_POINT('',#10869);
#2957=VERTEX_POINT('',#10871);
#2958=VERTEX_POINT('',#10873);
#2959=VERTEX_POINT('',#10875);
#2960=VERTEX_POINT('',#10877);
#2961=VERTEX_POINT('',#10879);
#2962=VERTEX_POINT('',#10881);
#2963=VERTEX_POINT('',#10883);
#2964=VERTEX_POINT('',#10885);
#2965=VERTEX_POINT('',#10887);
#2966=VERTEX_POINT('',#10889);
#2967=VERTEX_POINT('',#10891);
#2968=VERTEX_POINT('',#10893);
#2969=VERTEX_POINT('',#10895);
#2970=VERTEX_POINT('',#10897);
#2971=VERTEX_POINT('',#10899);
#2972=VERTEX_POINT('',#10901);
#2973=VERTEX_POINT('',#10903);
#2974=VERTEX_POINT('',#10905);
#2975=VERTEX_POINT('',#10907);
#2976=VERTEX_POINT('',#10909);
#2977=VERTEX_POINT('',#10911);
#2978=VERTEX_POINT('',#10913);
#2979=VERTEX_POINT('',#10915);
#2980=VERTEX_POINT('',#10917);
#2981=VERTEX_POINT('',#10919);
#2982=VERTEX_POINT('',#10921);
#2983=VERTEX_POINT('',#10923);
#2984=VERTEX_POINT('',#10925);
#2985=VERTEX_POINT('',#10927);
#2986=VERTEX_POINT('',#10929);
#2987=VERTEX_POINT('',#10931);
#2988=VERTEX_POINT('',#10933);
#2989=VERTEX_POINT('',#10935);
#2990=VERTEX_POINT('',#10937);
#2991=VERTEX_POINT('',#10939);
#2992=VERTEX_POINT('',#10941);
#2993=VERTEX_POINT('',#10943);
#2994=VERTEX_POINT('',#10945);
#2995=VERTEX_POINT('',#10947);
#2996=VERTEX_POINT('',#10949);
#2997=VERTEX_POINT('',#10951);
#2998=VERTEX_POINT('',#10953);
#2999=VERTEX_POINT('',#10955);
#3000=VERTEX_POINT('',#10957);
#3001=VERTEX_POINT('',#10959);
#3002=VERTEX_POINT('',#10961);
#3003=VERTEX_POINT('',#10963);
#3004=VERTEX_POINT('',#10965);
#3005=VERTEX_POINT('',#10967);
#3006=VERTEX_POINT('',#10969);
#3007=VERTEX_POINT('',#10971);
#3008=VERTEX_POINT('',#10973);
#3009=VERTEX_POINT('',#10975);
#3010=VERTEX_POINT('',#10977);
#3011=VERTEX_POINT('',#10979);
#3012=VERTEX_POINT('',#10981);
#3013=VERTEX_POINT('',#10983);
#3014=VERTEX_POINT('',#10985);
#3015=VERTEX_POINT('',#10987);
#3016=VERTEX_POINT('',#10989);
#3017=VERTEX_POINT('',#10991);
#3018=VERTEX_POINT('',#10993);
#3019=VERTEX_POINT('',#10995);
#3020=VERTEX_POINT('',#10997);
#3021=VERTEX_POINT('',#10999);
#3022=VERTEX_POINT('',#11001);
#3023=VERTEX_POINT('',#11003);
#3024=VERTEX_POINT('',#11005);
#3025=VERTEX_POINT('',#11009);
#3026=VERTEX_POINT('',#11014);
#3027=VERTEX_POINT('',#11016);
#3028=VERTEX_POINT('',#11017);
#3029=VERTEX_POINT('',#11019);
#3030=VERTEX_POINT('',#11021);
#3031=VERTEX_POINT('',#11023);
#3032=VERTEX_POINT('',#11025);
#3033=VERTEX_POINT('',#11027);
#3034=VERTEX_POINT('',#11029);
#3035=VERTEX_POINT('',#11031);
#3036=VERTEX_POINT('',#11033);
#3037=VERTEX_POINT('',#11035);
#3038=VERTEX_POINT('',#11037);
#3039=VERTEX_POINT('',#11039);
#3040=VERTEX_POINT('',#11041);
#3041=VERTEX_POINT('',#11043);
#3042=VERTEX_POINT('',#11045);
#3043=VERTEX_POINT('',#11047);
#3044=VERTEX_POINT('',#11049);
#3045=VERTEX_POINT('',#11051);
#3046=VERTEX_POINT('',#11053);
#3047=VERTEX_POINT('',#11055);
#3048=VERTEX_POINT('',#11057);
#3049=VERTEX_POINT('',#11059);
#3050=VERTEX_POINT('',#11061);
#3051=VERTEX_POINT('',#11063);
#3052=VERTEX_POINT('',#11065);
#3053=VERTEX_POINT('',#11067);
#3054=VERTEX_POINT('',#11069);
#3055=VERTEX_POINT('',#11071);
#3056=VERTEX_POINT('',#11073);
#3057=VERTEX_POINT('',#11075);
#3058=VERTEX_POINT('',#11077);
#3059=VERTEX_POINT('',#11079);
#3060=VERTEX_POINT('',#11081);
#3061=VERTEX_POINT('',#11083);
#3062=VERTEX_POINT('',#11085);
#3063=VERTEX_POINT('',#11087);
#3064=VERTEX_POINT('',#11089);
#3065=VERTEX_POINT('',#11091);
#3066=VERTEX_POINT('',#11093);
#3067=VERTEX_POINT('',#11095);
#3068=VERTEX_POINT('',#11097);
#3069=VERTEX_POINT('',#11099);
#3070=VERTEX_POINT('',#11101);
#3071=VERTEX_POINT('',#11103);
#3072=VERTEX_POINT('',#11105);
#3073=VERTEX_POINT('',#11107);
#3074=VERTEX_POINT('',#11109);
#3075=VERTEX_POINT('',#11111);
#3076=VERTEX_POINT('',#11113);
#3077=VERTEX_POINT('',#11115);
#3078=VERTEX_POINT('',#11117);
#3079=VERTEX_POINT('',#11119);
#3080=VERTEX_POINT('',#11121);
#3081=VERTEX_POINT('',#11123);
#3082=VERTEX_POINT('',#11125);
#3083=VERTEX_POINT('',#11127);
#3084=VERTEX_POINT('',#11129);
#3085=VERTEX_POINT('',#11131);
#3086=VERTEX_POINT('',#11133);
#3087=VERTEX_POINT('',#11135);
#3088=VERTEX_POINT('',#11137);
#3089=VERTEX_POINT('',#11139);
#3090=VERTEX_POINT('',#11141);
#3091=VERTEX_POINT('',#11143);
#3092=VERTEX_POINT('',#11145);
#3093=VERTEX_POINT('',#11147);
#3094=VERTEX_POINT('',#11149);
#3095=VERTEX_POINT('',#11151);
#3096=VERTEX_POINT('',#11153);
#3097=VERTEX_POINT('',#11155);
#3098=VERTEX_POINT('',#11157);
#3099=VERTEX_POINT('',#11159);
#3100=VERTEX_POINT('',#11161);
#3101=VERTEX_POINT('',#11163);
#3102=VERTEX_POINT('',#11165);
#3103=VERTEX_POINT('',#11167);
#3104=VERTEX_POINT('',#11169);
#3105=VERTEX_POINT('',#11171);
#3106=VERTEX_POINT('',#11173);
#3584=EDGE_CURVE('',#2914,#2915,#1699,.T.);
#3585=EDGE_CURVE('',#2914,#2916,#1700,.T.);
#3586=EDGE_CURVE('',#2917,#2916,#1701,.T.);
#3587=EDGE_CURVE('',#2915,#2917,#1702,.T.);
#3588=EDGE_CURVE('',#2918,#2914,#1703,.T.);
#3589=EDGE_CURVE('',#2918,#2919,#1704,.T.);
#3590=EDGE_CURVE('',#2916,#2919,#1705,.T.);
#3591=EDGE_CURVE('',#2920,#2920,#2460,.T.);
#3592=EDGE_CURVE('',#2921,#2918,#1706,.T.);
#3593=EDGE_CURVE('',#2922,#2921,#1707,.T.);
#3594=EDGE_CURVE('',#2919,#2922,#1708,.T.);
#3595=EDGE_CURVE('',#2923,#2923,#2461,.T.);
#3596=EDGE_CURVE('',#2922,#2917,#2462,.T.);
#3597=EDGE_CURVE('',#2915,#2921,#2463,.T.);
#3598=EDGE_CURVE('',#2924,#2925,#243,.T.);
#3599=EDGE_CURVE('',#2925,#2924,#244,.T.);
#3600=EDGE_CURVE('',#2926,#2927,#245,.T.);
#3601=EDGE_CURVE('',#2927,#2926,#246,.T.);
#3602=EDGE_CURVE('',#2928,#2929,#247,.T.);
#3603=EDGE_CURVE('',#2929,#2928,#248,.T.);
#3604=EDGE_CURVE('',#2930,#2931,#249,.T.);
#3605=EDGE_CURVE('',#2932,#2930,#250,.T.);
#3606=EDGE_CURVE('',#2931,#2932,#251,.T.);
#3607=EDGE_CURVE('',#2931,#2927,#1709,.T.);
#3608=EDGE_CURVE('',#2929,#2933,#1710,.T.);
#3609=EDGE_CURVE('',#2934,#2933,#252,.T.);
#3610=EDGE_CURVE('',#2935,#2934,#253,.T.);
#3611=EDGE_CURVE('',#2933,#2935,#254,.T.);
#3612=EDGE_CURVE('',#2936,#2936,#2464,.T.);
#3613=EDGE_CURVE('',#2936,#2932,#1711,.T.);
#3614=EDGE_CURVE('',#2930,#2937,#1712,.T.);
#3615=EDGE_CURVE('',#2937,#2937,#2465,.T.);
#3616=EDGE_CURVE('',#2938,#2939,#255,.T.);
#3617=EDGE_CURVE('',#2939,#2940,#256,.T.);
#3618=EDGE_CURVE('',#2940,#2938,#257,.T.);
#3619=EDGE_CURVE('',#2941,#2942,#258,.T.);
#3620=EDGE_CURVE('',#2942,#2943,#259,.T.);
#3621=EDGE_CURVE('',#2943,#2941,#260,.T.);
#3622=EDGE_CURVE('',#2940,#2920,#1713,.T.);
#3623=EDGE_CURVE('',#2925,#2943,#1714,.T.);
#3624=EDGE_CURVE('',#2944,#2944,#2466,.T.);
#3625=EDGE_CURVE('',#2945,#2946,#2467,.T.);
#3626=EDGE_CURVE('',#2947,#2946,#2468,.T.);
#3627=EDGE_CURVE('',#2947,#2948,#2469,.T.);
#3628=EDGE_CURVE('',#2949,#2948,#2470,.T.);
#3629=EDGE_CURVE('',#2949,#2950,#2471,.T.);
#3630=EDGE_CURVE('',#2951,#2950,#2472,.T.);
#3631=EDGE_CURVE('',#2951,#2952,#2473,.T.);
#3632=EDGE_CURVE('',#2953,#2952,#2474,.T.);
#3633=EDGE_CURVE('',#2953,#2954,#2475,.T.);
#3634=EDGE_CURVE('',#2955,#2954,#2476,.T.);
#3635=EDGE_CURVE('',#2955,#2956,#2477,.T.);
#3636=EDGE_CURVE('',#2957,#2956,#2478,.T.);
#3637=EDGE_CURVE('',#2957,#2958,#2479,.T.);
#3638=EDGE_CURVE('',#2959,#2958,#2480,.T.);
#3639=EDGE_CURVE('',#2959,#2960,#2481,.T.);
#3640=EDGE_CURVE('',#2961,#2960,#2482,.T.);
#3641=EDGE_CURVE('',#2961,#2962,#2483,.T.);
#3642=EDGE_CURVE('',#2963,#2962,#2484,.T.);
#3643=EDGE_CURVE('',#2963,#2964,#2485,.T.);
#3644=EDGE_CURVE('',#2965,#2964,#2486,.T.);
#3645=EDGE_CURVE('',#2965,#2966,#2487,.T.);
#3646=EDGE_CURVE('',#2967,#2966,#2488,.T.);
#3647=EDGE_CURVE('',#2967,#2968,#2489,.T.);
#3648=EDGE_CURVE('',#2969,#2968,#2490,.T.);
#3649=EDGE_CURVE('',#2969,#2970,#2491,.T.);
#3650=EDGE_CURVE('',#2971,#2970,#2492,.T.);
#3651=EDGE_CURVE('',#2971,#2972,#2493,.T.);
#3652=EDGE_CURVE('',#2973,#2972,#2494,.T.);
#3653=EDGE_CURVE('',#2973,#2974,#2495,.T.);
#3654=EDGE_CURVE('',#2975,#2974,#2496,.T.);
#3655=EDGE_CURVE('',#2975,#2976,#2497,.T.);
#3656=EDGE_CURVE('',#2977,#2976,#2498,.T.);
#3657=EDGE_CURVE('',#2977,#2978,#2499,.T.);
#3658=EDGE_CURVE('',#2979,#2978,#2500,.T.);
#3659=EDGE_CURVE('',#2979,#2980,#2501,.T.);
#3660=EDGE_CURVE('',#2981,#2980,#2502,.T.);
#3661=EDGE_CURVE('',#2981,#2982,#2503,.T.);
#3662=EDGE_CURVE('',#2983,#2982,#2504,.T.);
#3663=EDGE_CURVE('',#2983,#2984,#2505,.T.);
#3664=EDGE_CURVE('',#2985,#2984,#2506,.T.);
#3665=EDGE_CURVE('',#2985,#2986,#2507,.T.);
#3666=EDGE_CURVE('',#2987,#2986,#2508,.T.);
#3667=EDGE_CURVE('',#2987,#2988,#2509,.T.);
#3668=EDGE_CURVE('',#2989,#2988,#2510,.T.);
#3669=EDGE_CURVE('',#2989,#2990,#2511,.T.);
#3670=EDGE_CURVE('',#2991,#2990,#2512,.T.);
#3671=EDGE_CURVE('',#2991,#2992,#2513,.T.);
#3672=EDGE_CURVE('',#2993,#2992,#2514,.T.);
#3673=EDGE_CURVE('',#2993,#2994,#2515,.T.);
#3674=EDGE_CURVE('',#2995,#2994,#2516,.T.);
#3675=EDGE_CURVE('',#2995,#2996,#2517,.T.);
#3676=EDGE_CURVE('',#2997,#2996,#2518,.T.);
#3677=EDGE_CURVE('',#2997,#2998,#2519,.T.);
#3678=EDGE_CURVE('',#2999,#2998,#2520,.T.);
#3679=EDGE_CURVE('',#2999,#3000,#2521,.T.);
#3680=EDGE_CURVE('',#3001,#3000,#2522,.T.);
#3681=EDGE_CURVE('',#3001,#3002,#2523,.T.);
#3682=EDGE_CURVE('',#3003,#3002,#2524,.T.);
#3683=EDGE_CURVE('',#3003,#3004,#2525,.T.);
#3684=EDGE_CURVE('',#3005,#3004,#2526,.T.);
#3685=EDGE_CURVE('',#3005,#3006,#2527,.T.);
#3686=EDGE_CURVE('',#3007,#3006,#2528,.T.);
#3687=EDGE_CURVE('',#3007,#3008,#2529,.T.);
#3688=EDGE_CURVE('',#3009,#3008,#2530,.T.);
#3689=EDGE_CURVE('',#3009,#3010,#2531,.T.);
#3690=EDGE_CURVE('',#3011,#3010,#2532,.T.);
#3691=EDGE_CURVE('',#3011,#3012,#2533,.T.);
#3692=EDGE_CURVE('',#3013,#3012,#2534,.T.);
#3693=EDGE_CURVE('',#3013,#3014,#2535,.T.);
#3694=EDGE_CURVE('',#3015,#3014,#2536,.T.);
#3695=EDGE_CURVE('',#3015,#3016,#2537,.T.);
#3696=EDGE_CURVE('',#3017,#3016,#2538,.T.);
#3697=EDGE_CURVE('',#3017,#3018,#2539,.T.);
#3698=EDGE_CURVE('',#3019,#3018,#2540,.T.);
#3699=EDGE_CURVE('',#3019,#3020,#2541,.T.);
#3700=EDGE_CURVE('',#3021,#3020,#2542,.T.);
#3701=EDGE_CURVE('',#3021,#3022,#2543,.T.);
#3702=EDGE_CURVE('',#3023,#3022,#2544,.T.);
#3703=EDGE_CURVE('',#3023,#3024,#2545,.T.);
#3704=EDGE_CURVE('',#2945,#3024,#2546,.T.);
#3705=EDGE_CURVE('',#3025,#3025,#2547,.T.);
#3706=EDGE_CURVE('',#3025,#2944,#1715,.T.);
#3707=EDGE_CURVE('',#3026,#3026,#2548,.T.);
#3708=EDGE_CURVE('',#3027,#3028,#2549,.T.);
#3709=EDGE_CURVE('',#3028,#3029,#2550,.T.);
#3710=EDGE_CURVE('',#3029,#3030,#2551,.T.);
#3711=EDGE_CURVE('',#3030,#3031,#2552,.T.);
#3712=EDGE_CURVE('',#3031,#3032,#2553,.T.);
#3713=EDGE_CURVE('',#3032,#3033,#2554,.T.);
#3714=EDGE_CURVE('',#3033,#3034,#2555,.T.);
#3715=EDGE_CURVE('',#3034,#3035,#2556,.T.);
#3716=EDGE_CURVE('',#3035,#3036,#2557,.T.);
#3717=EDGE_CURVE('',#3036,#3037,#2558,.T.);
#3718=EDGE_CURVE('',#3037,#3038,#2559,.T.);
#3719=EDGE_CURVE('',#3038,#3039,#2560,.T.);
#3720=EDGE_CURVE('',#3039,#3040,#2561,.T.);
#3721=EDGE_CURVE('',#3040,#3041,#2562,.T.);
#3722=EDGE_CURVE('',#3041,#3042,#2563,.T.);
#3723=EDGE_CURVE('',#3042,#3043,#2564,.T.);
#3724=EDGE_CURVE('',#3043,#3044,#2565,.T.);
#3725=EDGE_CURVE('',#3044,#3045,#2566,.T.);
#3726=EDGE_CURVE('',#3045,#3046,#2567,.T.);
#3727=EDGE_CURVE('',#3046,#3047,#2568,.T.);
#3728=EDGE_CURVE('',#3047,#3048,#2569,.T.);
#3729=EDGE_CURVE('',#3048,#3049,#2570,.T.);
#3730=EDGE_CURVE('',#3049,#3050,#2571,.T.);
#3731=EDGE_CURVE('',#3050,#3051,#2572,.T.);
#3732=EDGE_CURVE('',#3051,#3052,#2573,.T.);
#3733=EDGE_CURVE('',#3052,#3053,#2574,.T.);
#3734=EDGE_CURVE('',#3053,#3054,#2575,.T.);
#3735=EDGE_CURVE('',#3054,#3055,#2576,.T.);
#3736=EDGE_CURVE('',#3055,#3056,#2577,.T.);
#3737=EDGE_CURVE('',#3056,#3057,#2578,.T.);
#3738=EDGE_CURVE('',#3057,#3058,#2579,.T.);
#3739=EDGE_CURVE('',#3058,#3059,#2580,.T.);
#3740=EDGE_CURVE('',#3059,#3060,#2581,.T.);
#3741=EDGE_CURVE('',#3060,#3061,#2582,.T.);
#3742=EDGE_CURVE('',#3061,#3062,#2583,.T.);
#3743=EDGE_CURVE('',#3062,#3063,#2584,.T.);
#3744=EDGE_CURVE('',#3063,#3064,#2585,.T.);
#3745=EDGE_CURVE('',#3064,#3065,#2586,.T.);
#3746=EDGE_CURVE('',#3065,#3066,#2587,.T.);
#3747=EDGE_CURVE('',#3066,#3067,#2588,.T.);
#3748=EDGE_CURVE('',#3067,#3068,#2589,.T.);
#3749=EDGE_CURVE('',#3068,#3069,#2590,.T.);
#3750=EDGE_CURVE('',#3069,#3070,#2591,.T.);
#3751=EDGE_CURVE('',#3070,#3071,#2592,.T.);
#3752=EDGE_CURVE('',#3071,#3072,#2593,.T.);
#3753=EDGE_CURVE('',#3072,#3073,#2594,.T.);
#3754=EDGE_CURVE('',#3073,#3074,#2595,.T.);
#3755=EDGE_CURVE('',#3074,#3075,#2596,.T.);
#3756=EDGE_CURVE('',#3075,#3076,#2597,.T.);
#3757=EDGE_CURVE('',#3076,#3077,#2598,.T.);
#3758=EDGE_CURVE('',#3077,#3078,#2599,.T.);
#3759=EDGE_CURVE('',#3078,#3079,#2600,.T.);
#3760=EDGE_CURVE('',#3079,#3080,#2601,.T.);
#3761=EDGE_CURVE('',#3080,#3081,#2602,.T.);
#3762=EDGE_CURVE('',#3081,#3082,#2603,.T.);
#3763=EDGE_CURVE('',#3082,#3083,#2604,.T.);
#3764=EDGE_CURVE('',#3083,#3084,#2605,.T.);
#3765=EDGE_CURVE('',#3084,#3085,#2606,.T.);
#3766=EDGE_CURVE('',#3085,#3086,#2607,.T.);
#3767=EDGE_CURVE('',#3086,#3087,#2608,.T.);
#3768=EDGE_CURVE('',#3087,#3088,#2609,.T.);
#3769=EDGE_CURVE('',#3088,#3089,#2610,.T.);
#3770=EDGE_CURVE('',#3089,#3090,#2611,.T.);
#3771=EDGE_CURVE('',#3090,#3091,#2612,.T.);
#3772=EDGE_CURVE('',#3091,#3092,#2613,.T.);
#3773=EDGE_CURVE('',#3092,#3093,#2614,.T.);
#3774=EDGE_CURVE('',#3093,#3094,#2615,.T.);
#3775=EDGE_CURVE('',#3094,#3095,#2616,.T.);
#3776=EDGE_CURVE('',#3095,#3096,#2617,.T.);
#3777=EDGE_CURVE('',#3096,#3097,#2618,.T.);
#3778=EDGE_CURVE('',#3097,#3098,#2619,.T.);
#3779=EDGE_CURVE('',#3098,#3099,#2620,.T.);
#3780=EDGE_CURVE('',#3099,#3100,#2621,.T.);
#3781=EDGE_CURVE('',#3100,#3101,#2622,.T.);
#3782=EDGE_CURVE('',#3101,#3102,#2623,.T.);
#3783=EDGE_CURVE('',#3102,#3103,#2624,.T.);
#3784=EDGE_CURVE('',#3103,#3104,#2625,.T.);
#3785=EDGE_CURVE('',#3104,#3105,#2626,.T.);
#3786=EDGE_CURVE('',#3105,#3106,#2627,.T.);
#3787=EDGE_CURVE('',#3106,#3027,#2628,.T.);
#3788=EDGE_CURVE('',#2923,#3026,#1716,.T.);
#3789=EDGE_CURVE('',#3028,#2945,#1717,.T.);
#3790=EDGE_CURVE('',#2946,#3027,#1718,.T.);
#3791=EDGE_CURVE('',#3106,#2947,#1719,.T.);
#3792=EDGE_CURVE('',#2948,#3105,#1720,.T.);
#3793=EDGE_CURVE('',#3104,#2949,#1721,.T.);
#3794=EDGE_CURVE('',#2950,#3103,#1722,.T.);
#3795=EDGE_CURVE('',#3102,#2951,#1723,.T.);
#3796=EDGE_CURVE('',#2952,#3101,#1724,.T.);
#3797=EDGE_CURVE('',#3100,#2953,#1725,.T.);
#3798=EDGE_CURVE('',#2954,#3099,#1726,.T.);
#3799=EDGE_CURVE('',#3098,#2955,#1727,.T.);
#3800=EDGE_CURVE('',#2956,#3097,#1728,.T.);
#3801=EDGE_CURVE('',#3096,#2957,#1729,.T.);
#3802=EDGE_CURVE('',#2958,#3095,#1730,.T.);
#3803=EDGE_CURVE('',#3094,#2959,#1731,.T.);
#3804=EDGE_CURVE('',#2960,#3093,#1732,.T.);
#3805=EDGE_CURVE('',#3092,#2961,#1733,.T.);
#3806=EDGE_CURVE('',#2962,#3091,#1734,.T.);
#3807=EDGE_CURVE('',#3090,#2963,#1735,.T.);
#3808=EDGE_CURVE('',#2964,#3089,#1736,.T.);
#3809=EDGE_CURVE('',#3088,#2965,#1737,.T.);
#3810=EDGE_CURVE('',#2966,#3087,#1738,.T.);
#3811=EDGE_CURVE('',#3086,#2967,#1739,.T.);
#3812=EDGE_CURVE('',#2968,#3085,#1740,.T.);
#3813=EDGE_CURVE('',#3084,#2969,#1741,.T.);
#3814=EDGE_CURVE('',#2970,#3083,#1742,.T.);
#3815=EDGE_CURVE('',#3082,#2971,#1743,.T.);
#3816=EDGE_CURVE('',#2972,#3081,#1744,.T.);
#3817=EDGE_CURVE('',#3080,#2973,#1745,.T.);
#3818=EDGE_CURVE('',#2974,#3079,#1746,.T.);
#3819=EDGE_CURVE('',#3078,#2975,#1747,.T.);
#3820=EDGE_CURVE('',#2976,#3077,#1748,.T.);
#3821=EDGE_CURVE('',#3076,#2977,#1749,.T.);
#3822=EDGE_CURVE('',#2978,#3075,#1750,.T.);
#3823=EDGE_CURVE('',#3074,#2979,#1751,.T.);
#3824=EDGE_CURVE('',#2980,#3073,#1752,.T.);
#3825=EDGE_CURVE('',#3072,#2981,#1753,.T.);
#3826=EDGE_CURVE('',#2982,#3071,#1754,.T.);
#3827=EDGE_CURVE('',#3070,#2983,#1755,.T.);
#3828=EDGE_CURVE('',#2984,#3069,#1756,.T.);
#3829=EDGE_CURVE('',#3068,#2985,#1757,.T.);
#3830=EDGE_CURVE('',#2986,#3067,#1758,.T.);
#3831=EDGE_CURVE('',#3066,#2987,#1759,.T.);
#3832=EDGE_CURVE('',#2988,#3065,#1760,.T.);
#3833=EDGE_CURVE('',#3064,#2989,#1761,.T.);
#3834=EDGE_CURVE('',#2990,#3063,#1762,.T.);
#3835=EDGE_CURVE('',#3062,#2991,#1763,.T.);
#3836=EDGE_CURVE('',#2992,#3061,#1764,.T.);
#3837=EDGE_CURVE('',#3060,#2993,#1765,.T.);
#3838=EDGE_CURVE('',#2994,#3059,#1766,.T.);
#3839=EDGE_CURVE('',#3058,#2995,#1767,.T.);
#3840=EDGE_CURVE('',#2996,#3057,#1768,.T.);
#3841=EDGE_CURVE('',#3056,#2997,#1769,.T.);
#3842=EDGE_CURVE('',#2998,#3055,#1770,.T.);
#3843=EDGE_CURVE('',#3054,#2999,#1771,.T.);
#3844=EDGE_CURVE('',#3000,#3053,#1772,.T.);
#3845=EDGE_CURVE('',#3052,#3001,#1773,.T.);
#3846=EDGE_CURVE('',#3002,#3051,#1774,.T.);
#3847=EDGE_CURVE('',#3050,#3003,#1775,.T.);
#3848=EDGE_CURVE('',#3004,#3049,#1776,.T.);
#3849=EDGE_CURVE('',#3048,#3005,#1777,.T.);
#3850=EDGE_CURVE('',#3006,#3047,#1778,.T.);
#3851=EDGE_CURVE('',#3046,#3007,#1779,.T.);
#3852=EDGE_CURVE('',#3008,#3045,#1780,.T.);
#3853=EDGE_CURVE('',#3044,#3009,#1781,.T.);
#3854=EDGE_CURVE('',#3010,#3043,#1782,.T.);
#3855=EDGE_CURVE('',#3042,#3011,#1783,.T.);
#3856=EDGE_CURVE('',#3012,#3041,#1784,.T.);
#3857=EDGE_CURVE('',#3040,#3013,#1785,.T.);
#3858=EDGE_CURVE('',#3014,#3039,#1786,.T.);
#3859=EDGE_CURVE('',#3038,#3015,#1787,.T.);
#3860=EDGE_CURVE('',#3016,#3037,#1788,.T.);
#3861=EDGE_CURVE('',#3036,#3017,#1789,.T.);
#3862=EDGE_CURVE('',#3018,#3035,#1790,.T.);
#3863=EDGE_CURVE('',#3034,#3019,#1791,.T.);
#3864=EDGE_CURVE('',#3020,#3033,#1792,.T.);
#3865=EDGE_CURVE('',#3032,#3021,#1793,.T.);
#3866=EDGE_CURVE('',#3022,#3031,#1794,.T.);
#3867=EDGE_CURVE('',#3024,#3029,#1795,.T.);
#3868=EDGE_CURVE('',#3030,#3023,#1796,.T.);
#4783=ORIENTED_EDGE('',*,*,#3584,.F.);
#4784=ORIENTED_EDGE('',*,*,#3585,.T.);
#4785=ORIENTED_EDGE('',*,*,#3586,.F.);
#4786=ORIENTED_EDGE('',*,*,#3587,.F.);
#4787=ORIENTED_EDGE('',*,*,#3588,.F.);
#4788=ORIENTED_EDGE('',*,*,#3589,.T.);
#4789=ORIENTED_EDGE('',*,*,#3590,.F.);
#4790=ORIENTED_EDGE('',*,*,#3585,.F.);
#4791=ORIENTED_EDGE('',*,*,#3591,.F.);
#4792=ORIENTED_EDGE('',*,*,#3592,.F.);
#4793=ORIENTED_EDGE('',*,*,#3593,.F.);
#4794=ORIENTED_EDGE('',*,*,#3594,.F.);
#4795=ORIENTED_EDGE('',*,*,#3589,.F.);
#4796=ORIENTED_EDGE('',*,*,#3595,.T.);
#4797=ORIENTED_EDGE('',*,*,#3586,.T.);
#4798=ORIENTED_EDGE('',*,*,#3590,.T.);
#4799=ORIENTED_EDGE('',*,*,#3594,.T.);
#4800=ORIENTED_EDGE('',*,*,#3596,.T.);
#4801=ORIENTED_EDGE('',*,*,#3587,.T.);
#4802=ORIENTED_EDGE('',*,*,#3596,.F.);
#4803=ORIENTED_EDGE('',*,*,#3593,.T.);
#4804=ORIENTED_EDGE('',*,*,#3597,.F.);
#4805=ORIENTED_EDGE('',*,*,#3598,.T.);
#4806=ORIENTED_EDGE('',*,*,#3599,.T.);
#4807=ORIENTED_EDGE('',*,*,#3600,.T.);
#4808=ORIENTED_EDGE('',*,*,#3601,.T.);
#4809=ORIENTED_EDGE('',*,*,#3602,.T.);
#4810=ORIENTED_EDGE('',*,*,#3603,.T.);
#4811=ORIENTED_EDGE('',*,*,#3604,.F.);
#4812=ORIENTED_EDGE('',*,*,#3605,.F.);
#4813=ORIENTED_EDGE('',*,*,#3606,.F.);
#4814=ORIENTED_EDGE('',*,*,#3607,.T.);
#4815=ORIENTED_EDGE('',*,*,#3600,.F.);
#4816=ORIENTED_EDGE('',*,*,#3601,.F.);
#4817=ORIENTED_EDGE('',*,*,#3607,.F.);
#4818=ORIENTED_EDGE('',*,*,#3602,.F.);
#4819=ORIENTED_EDGE('',*,*,#3603,.F.);
#4820=ORIENTED_EDGE('',*,*,#3608,.T.);
#4821=ORIENTED_EDGE('',*,*,#3609,.F.);
#4822=ORIENTED_EDGE('',*,*,#3610,.F.);
#4823=ORIENTED_EDGE('',*,*,#3611,.F.);
#4824=ORIENTED_EDGE('',*,*,#3608,.F.);
#4825=ORIENTED_EDGE('',*,*,#3612,.F.);
#4826=ORIENTED_EDGE('',*,*,#3613,.T.);
#4827=ORIENTED_EDGE('',*,*,#3605,.T.);
#4828=ORIENTED_EDGE('',*,*,#3614,.T.);
#4829=ORIENTED_EDGE('',*,*,#3615,.F.);
#4830=ORIENTED_EDGE('',*,*,#3614,.F.);
#4831=ORIENTED_EDGE('',*,*,#3604,.T.);
#4832=ORIENTED_EDGE('',*,*,#3606,.T.);
#4833=ORIENTED_EDGE('',*,*,#3613,.F.);
#4834=ORIENTED_EDGE('',*,*,#3610,.T.);
#4835=ORIENTED_EDGE('',*,*,#3609,.T.);
#4836=ORIENTED_EDGE('',*,*,#3611,.T.);
#4837=ORIENTED_EDGE('',*,*,#3616,.T.);
#4838=ORIENTED_EDGE('',*,*,#3617,.T.);
#4839=ORIENTED_EDGE('',*,*,#3618,.T.);
#4840=ORIENTED_EDGE('',*,*,#3619,.T.);
#4841=ORIENTED_EDGE('',*,*,#3620,.T.);
#4842=ORIENTED_EDGE('',*,*,#3621,.T.);
#4843=ORIENTED_EDGE('',*,*,#3617,.F.);
#4844=ORIENTED_EDGE('',*,*,#3616,.F.);
#4845=ORIENTED_EDGE('',*,*,#3618,.F.);
#4846=ORIENTED_EDGE('',*,*,#3622,.T.);
#4847=ORIENTED_EDGE('',*,*,#3591,.T.);
#4848=ORIENTED_EDGE('',*,*,#3622,.F.);
#4849=ORIENTED_EDGE('',*,*,#3598,.F.);
#4850=ORIENTED_EDGE('',*,*,#3599,.F.);
#4851=ORIENTED_EDGE('',*,*,#3623,.T.);
#4852=ORIENTED_EDGE('',*,*,#3620,.F.);
#4853=ORIENTED_EDGE('',*,*,#3619,.F.);
#4854=ORIENTED_EDGE('',*,*,#3621,.F.);
#4855=ORIENTED_EDGE('',*,*,#3623,.F.);
#4856=ORIENTED_EDGE('',*,*,#3612,.T.);
#4857=ORIENTED_EDGE('',*,*,#3584,.T.);
#4858=ORIENTED_EDGE('',*,*,#3597,.T.);
#4859=ORIENTED_EDGE('',*,*,#3592,.T.);
#4860=ORIENTED_EDGE('',*,*,#3588,.T.);
#4861=ORIENTED_EDGE('',*,*,#3624,.T.);
#4862=ORIENTED_EDGE('',*,*,#3625,.T.);
#4863=ORIENTED_EDGE('',*,*,#3626,.F.);
#4864=ORIENTED_EDGE('',*,*,#3627,.T.);
#4865=ORIENTED_EDGE('',*,*,#3628,.F.);
#4866=ORIENTED_EDGE('',*,*,#3629,.T.);
#4867=ORIENTED_EDGE('',*,*,#3630,.F.);
#4868=ORIENTED_EDGE('',*,*,#3631,.T.);
#4869=ORIENTED_EDGE('',*,*,#3632,.F.);
#4870=ORIENTED_EDGE('',*,*,#3633,.T.);
#4871=ORIENTED_EDGE('',*,*,#3634,.F.);
#4872=ORIENTED_EDGE('',*,*,#3635,.T.);
#4873=ORIENTED_EDGE('',*,*,#3636,.F.);
#4874=ORIENTED_EDGE('',*,*,#3637,.T.);
#4875=ORIENTED_EDGE('',*,*,#3638,.F.);
#4876=ORIENTED_EDGE('',*,*,#3639,.T.);
#4877=ORIENTED_EDGE('',*,*,#3640,.F.);
#4878=ORIENTED_EDGE('',*,*,#3641,.T.);
#4879=ORIENTED_EDGE('',*,*,#3642,.F.);
#4880=ORIENTED_EDGE('',*,*,#3643,.T.);
#4881=ORIENTED_EDGE('',*,*,#3644,.F.);
#4882=ORIENTED_EDGE('',*,*,#3645,.T.);
#4883=ORIENTED_EDGE('',*,*,#3646,.F.);
#4884=ORIENTED_EDGE('',*,*,#3647,.T.);
#4885=ORIENTED_EDGE('',*,*,#3648,.F.);
#4886=ORIENTED_EDGE('',*,*,#3649,.T.);
#4887=ORIENTED_EDGE('',*,*,#3650,.F.);
#4888=ORIENTED_EDGE('',*,*,#3651,.T.);
#4889=ORIENTED_EDGE('',*,*,#3652,.F.);
#4890=ORIENTED_EDGE('',*,*,#3653,.T.);
#4891=ORIENTED_EDGE('',*,*,#3654,.F.);
#4892=ORIENTED_EDGE('',*,*,#3655,.T.);
#4893=ORIENTED_EDGE('',*,*,#3656,.F.);
#4894=ORIENTED_EDGE('',*,*,#3657,.T.);
#4895=ORIENTED_EDGE('',*,*,#3658,.F.);
#4896=ORIENTED_EDGE('',*,*,#3659,.T.);
#4897=ORIENTED_EDGE('',*,*,#3660,.F.);
#4898=ORIENTED_EDGE('',*,*,#3661,.T.);
#4899=ORIENTED_EDGE('',*,*,#3662,.F.);
#4900=ORIENTED_EDGE('',*,*,#3663,.T.);
#4901=ORIENTED_EDGE('',*,*,#3664,.F.);
#4902=ORIENTED_EDGE('',*,*,#3665,.T.);
#4903=ORIENTED_EDGE('',*,*,#3666,.F.);
#4904=ORIENTED_EDGE('',*,*,#3667,.T.);
#4905=ORIENTED_EDGE('',*,*,#3668,.F.);
#4906=ORIENTED_EDGE('',*,*,#3669,.T.);
#4907=ORIENTED_EDGE('',*,*,#3670,.F.);
#4908=ORIENTED_EDGE('',*,*,#3671,.T.);
#4909=ORIENTED_EDGE('',*,*,#3672,.F.);
#4910=ORIENTED_EDGE('',*,*,#3673,.T.);
#4911=ORIENTED_EDGE('',*,*,#3674,.F.);
#4912=ORIENTED_EDGE('',*,*,#3675,.T.);
#4913=ORIENTED_EDGE('',*,*,#3676,.F.);
#4914=ORIENTED_EDGE('',*,*,#3677,.T.);
#4915=ORIENTED_EDGE('',*,*,#3678,.F.);
#4916=ORIENTED_EDGE('',*,*,#3679,.T.);
#4917=ORIENTED_EDGE('',*,*,#3680,.F.);
#4918=ORIENTED_EDGE('',*,*,#3681,.T.);
#4919=ORIENTED_EDGE('',*,*,#3682,.F.);
#4920=ORIENTED_EDGE('',*,*,#3683,.T.);
#4921=ORIENTED_EDGE('',*,*,#3684,.F.);
#4922=ORIENTED_EDGE('',*,*,#3685,.T.);
#4923=ORIENTED_EDGE('',*,*,#3686,.F.);
#4924=ORIENTED_EDGE('',*,*,#3687,.T.);
#4925=ORIENTED_EDGE('',*,*,#3688,.F.);
#4926=ORIENTED_EDGE('',*,*,#3689,.T.);
#4927=ORIENTED_EDGE('',*,*,#3690,.F.);
#4928=ORIENTED_EDGE('',*,*,#3691,.T.);
#4929=ORIENTED_EDGE('',*,*,#3692,.F.);
#4930=ORIENTED_EDGE('',*,*,#3693,.T.);
#4931=ORIENTED_EDGE('',*,*,#3694,.F.);
#4932=ORIENTED_EDGE('',*,*,#3695,.T.);
#4933=ORIENTED_EDGE('',*,*,#3696,.F.);
#4934=ORIENTED_EDGE('',*,*,#3697,.T.);
#4935=ORIENTED_EDGE('',*,*,#3698,.F.);
#4936=ORIENTED_EDGE('',*,*,#3699,.T.);
#4937=ORIENTED_EDGE('',*,*,#3700,.F.);
#4938=ORIENTED_EDGE('',*,*,#3701,.T.);
#4939=ORIENTED_EDGE('',*,*,#3702,.F.);
#4940=ORIENTED_EDGE('',*,*,#3703,.T.);
#4941=ORIENTED_EDGE('',*,*,#3704,.F.);
#4942=ORIENTED_EDGE('',*,*,#3705,.F.);
#4943=ORIENTED_EDGE('',*,*,#3706,.T.);
#4944=ORIENTED_EDGE('',*,*,#3624,.F.);
#4945=ORIENTED_EDGE('',*,*,#3706,.F.);
#4946=ORIENTED_EDGE('',*,*,#3705,.T.);
#4947=ORIENTED_EDGE('',*,*,#3615,.T.);
#4948=ORIENTED_EDGE('',*,*,#3707,.F.);
#4949=ORIENTED_EDGE('',*,*,#3708,.T.);
#4950=ORIENTED_EDGE('',*,*,#3709,.T.);
#4951=ORIENTED_EDGE('',*,*,#3710,.T.);
#4952=ORIENTED_EDGE('',*,*,#3711,.T.);
#4953=ORIENTED_EDGE('',*,*,#3712,.T.);
#4954=ORIENTED_EDGE('',*,*,#3713,.T.);
#4955=ORIENTED_EDGE('',*,*,#3714,.T.);
#4956=ORIENTED_EDGE('',*,*,#3715,.T.);
#4957=ORIENTED_EDGE('',*,*,#3716,.T.);
#4958=ORIENTED_EDGE('',*,*,#3717,.T.);
#4959=ORIENTED_EDGE('',*,*,#3718,.T.);
#4960=ORIENTED_EDGE('',*,*,#3719,.T.);
#4961=ORIENTED_EDGE('',*,*,#3720,.T.);
#4962=ORIENTED_EDGE('',*,*,#3721,.T.);
#4963=ORIENTED_EDGE('',*,*,#3722,.T.);
#4964=ORIENTED_EDGE('',*,*,#3723,.T.);
#4965=ORIENTED_EDGE('',*,*,#3724,.T.);
#4966=ORIENTED_EDGE('',*,*,#3725,.T.);
#4967=ORIENTED_EDGE('',*,*,#3726,.T.);
#4968=ORIENTED_EDGE('',*,*,#3727,.T.);
#4969=ORIENTED_EDGE('',*,*,#3728,.T.);
#4970=ORIENTED_EDGE('',*,*,#3729,.T.);
#4971=ORIENTED_EDGE('',*,*,#3730,.T.);
#4972=ORIENTED_EDGE('',*,*,#3731,.T.);
#4973=ORIENTED_EDGE('',*,*,#3732,.T.);
#4974=ORIENTED_EDGE('',*,*,#3733,.T.);
#4975=ORIENTED_EDGE('',*,*,#3734,.T.);
#4976=ORIENTED_EDGE('',*,*,#3735,.T.);
#4977=ORIENTED_EDGE('',*,*,#3736,.T.);
#4978=ORIENTED_EDGE('',*,*,#3737,.T.);
#4979=ORIENTED_EDGE('',*,*,#3738,.T.);
#4980=ORIENTED_EDGE('',*,*,#3739,.T.);
#4981=ORIENTED_EDGE('',*,*,#3740,.T.);
#4982=ORIENTED_EDGE('',*,*,#3741,.T.);
#4983=ORIENTED_EDGE('',*,*,#3742,.T.);
#4984=ORIENTED_EDGE('',*,*,#3743,.T.);
#4985=ORIENTED_EDGE('',*,*,#3744,.T.);
#4986=ORIENTED_EDGE('',*,*,#3745,.T.);
#4987=ORIENTED_EDGE('',*,*,#3746,.T.);
#4988=ORIENTED_EDGE('',*,*,#3747,.T.);
#4989=ORIENTED_EDGE('',*,*,#3748,.T.);
#4990=ORIENTED_EDGE('',*,*,#3749,.T.);
#4991=ORIENTED_EDGE('',*,*,#3750,.T.);
#4992=ORIENTED_EDGE('',*,*,#3751,.T.);
#4993=ORIENTED_EDGE('',*,*,#3752,.T.);
#4994=ORIENTED_EDGE('',*,*,#3753,.T.);
#4995=ORIENTED_EDGE('',*,*,#3754,.T.);
#4996=ORIENTED_EDGE('',*,*,#3755,.T.);
#4997=ORIENTED_EDGE('',*,*,#3756,.T.);
#4998=ORIENTED_EDGE('',*,*,#3757,.T.);
#4999=ORIENTED_EDGE('',*,*,#3758,.T.);
#5000=ORIENTED_EDGE('',*,*,#3759,.T.);
#5001=ORIENTED_EDGE('',*,*,#3760,.T.);
#5002=ORIENTED_EDGE('',*,*,#3761,.T.);
#5003=ORIENTED_EDGE('',*,*,#3762,.T.);
#5004=ORIENTED_EDGE('',*,*,#3763,.T.);
#5005=ORIENTED_EDGE('',*,*,#3764,.T.);
#5006=ORIENTED_EDGE('',*,*,#3765,.T.);
#5007=ORIENTED_EDGE('',*,*,#3766,.T.);
#5008=ORIENTED_EDGE('',*,*,#3767,.T.);
#5009=ORIENTED_EDGE('',*,*,#3768,.T.);
#5010=ORIENTED_EDGE('',*,*,#3769,.T.);
#5011=ORIENTED_EDGE('',*,*,#3770,.T.);
#5012=ORIENTED_EDGE('',*,*,#3771,.T.);
#5013=ORIENTED_EDGE('',*,*,#3772,.T.);
#5014=ORIENTED_EDGE('',*,*,#3773,.T.);
#5015=ORIENTED_EDGE('',*,*,#3774,.T.);
#5016=ORIENTED_EDGE('',*,*,#3775,.T.);
#5017=ORIENTED_EDGE('',*,*,#3776,.T.);
#5018=ORIENTED_EDGE('',*,*,#3777,.T.);
#5019=ORIENTED_EDGE('',*,*,#3778,.T.);
#5020=ORIENTED_EDGE('',*,*,#3779,.T.);
#5021=ORIENTED_EDGE('',*,*,#3780,.T.);
#5022=ORIENTED_EDGE('',*,*,#3781,.T.);
#5023=ORIENTED_EDGE('',*,*,#3782,.T.);
#5024=ORIENTED_EDGE('',*,*,#3783,.T.);
#5025=ORIENTED_EDGE('',*,*,#3784,.T.);
#5026=ORIENTED_EDGE('',*,*,#3785,.T.);
#5027=ORIENTED_EDGE('',*,*,#3786,.T.);
#5028=ORIENTED_EDGE('',*,*,#3787,.T.);
#5029=ORIENTED_EDGE('',*,*,#3595,.F.);
#5030=ORIENTED_EDGE('',*,*,#3788,.T.);
#5031=ORIENTED_EDGE('',*,*,#3707,.T.);
#5032=ORIENTED_EDGE('',*,*,#3788,.F.);
#5033=ORIENTED_EDGE('',*,*,#3789,.F.);
#5034=ORIENTED_EDGE('',*,*,#3708,.F.);
#5035=ORIENTED_EDGE('',*,*,#3790,.F.);
#5036=ORIENTED_EDGE('',*,*,#3625,.F.);
#5037=ORIENTED_EDGE('',*,*,#3790,.T.);
#5038=ORIENTED_EDGE('',*,*,#3787,.F.);
#5039=ORIENTED_EDGE('',*,*,#3791,.T.);
#5040=ORIENTED_EDGE('',*,*,#3626,.T.);
#5041=ORIENTED_EDGE('',*,*,#3791,.F.);
#5042=ORIENTED_EDGE('',*,*,#3786,.F.);
#5043=ORIENTED_EDGE('',*,*,#3792,.F.);
#5044=ORIENTED_EDGE('',*,*,#3627,.F.);
#5045=ORIENTED_EDGE('',*,*,#3792,.T.);
#5046=ORIENTED_EDGE('',*,*,#3785,.F.);
#5047=ORIENTED_EDGE('',*,*,#3793,.T.);
#5048=ORIENTED_EDGE('',*,*,#3628,.T.);
#5049=ORIENTED_EDGE('',*,*,#3793,.F.);
#5050=ORIENTED_EDGE('',*,*,#3784,.F.);
#5051=ORIENTED_EDGE('',*,*,#3794,.F.);
#5052=ORIENTED_EDGE('',*,*,#3629,.F.);
#5053=ORIENTED_EDGE('',*,*,#3794,.T.);
#5054=ORIENTED_EDGE('',*,*,#3783,.F.);
#5055=ORIENTED_EDGE('',*,*,#3795,.T.);
#5056=ORIENTED_EDGE('',*,*,#3630,.T.);
#5057=ORIENTED_EDGE('',*,*,#3795,.F.);
#5058=ORIENTED_EDGE('',*,*,#3782,.F.);
#5059=ORIENTED_EDGE('',*,*,#3796,.F.);
#5060=ORIENTED_EDGE('',*,*,#3631,.F.);
#5061=ORIENTED_EDGE('',*,*,#3796,.T.);
#5062=ORIENTED_EDGE('',*,*,#3781,.F.);
#5063=ORIENTED_EDGE('',*,*,#3797,.T.);
#5064=ORIENTED_EDGE('',*,*,#3632,.T.);
#5065=ORIENTED_EDGE('',*,*,#3797,.F.);
#5066=ORIENTED_EDGE('',*,*,#3780,.F.);
#5067=ORIENTED_EDGE('',*,*,#3798,.F.);
#5068=ORIENTED_EDGE('',*,*,#3633,.F.);
#5069=ORIENTED_EDGE('',*,*,#3798,.T.);
#5070=ORIENTED_EDGE('',*,*,#3779,.F.);
#5071=ORIENTED_EDGE('',*,*,#3799,.T.);
#5072=ORIENTED_EDGE('',*,*,#3634,.T.);
#5073=ORIENTED_EDGE('',*,*,#3799,.F.);
#5074=ORIENTED_EDGE('',*,*,#3778,.F.);
#5075=ORIENTED_EDGE('',*,*,#3800,.F.);
#5076=ORIENTED_EDGE('',*,*,#3635,.F.);
#5077=ORIENTED_EDGE('',*,*,#3800,.T.);
#5078=ORIENTED_EDGE('',*,*,#3777,.F.);
#5079=ORIENTED_EDGE('',*,*,#3801,.T.);
#5080=ORIENTED_EDGE('',*,*,#3636,.T.);
#5081=ORIENTED_EDGE('',*,*,#3801,.F.);
#5082=ORIENTED_EDGE('',*,*,#3776,.F.);
#5083=ORIENTED_EDGE('',*,*,#3802,.F.);
#5084=ORIENTED_EDGE('',*,*,#3637,.F.);
#5085=ORIENTED_EDGE('',*,*,#3802,.T.);
#5086=ORIENTED_EDGE('',*,*,#3775,.F.);
#5087=ORIENTED_EDGE('',*,*,#3803,.T.);
#5088=ORIENTED_EDGE('',*,*,#3638,.T.);
#5089=ORIENTED_EDGE('',*,*,#3803,.F.);
#5090=ORIENTED_EDGE('',*,*,#3774,.F.);
#5091=ORIENTED_EDGE('',*,*,#3804,.F.);
#5092=ORIENTED_EDGE('',*,*,#3639,.F.);
#5093=ORIENTED_EDGE('',*,*,#3804,.T.);
#5094=ORIENTED_EDGE('',*,*,#3773,.F.);
#5095=ORIENTED_EDGE('',*,*,#3805,.T.);
#5096=ORIENTED_EDGE('',*,*,#3640,.T.);
#5097=ORIENTED_EDGE('',*,*,#3805,.F.);
#5098=ORIENTED_EDGE('',*,*,#3772,.F.);
#5099=ORIENTED_EDGE('',*,*,#3806,.F.);
#5100=ORIENTED_EDGE('',*,*,#3641,.F.);
#5101=ORIENTED_EDGE('',*,*,#3806,.T.);
#5102=ORIENTED_EDGE('',*,*,#3771,.F.);
#5103=ORIENTED_EDGE('',*,*,#3807,.T.);
#5104=ORIENTED_EDGE('',*,*,#3642,.T.);
#5105=ORIENTED_EDGE('',*,*,#3807,.F.);
#5106=ORIENTED_EDGE('',*,*,#3770,.F.);
#5107=ORIENTED_EDGE('',*,*,#3808,.F.);
#5108=ORIENTED_EDGE('',*,*,#3643,.F.);
#5109=ORIENTED_EDGE('',*,*,#3808,.T.);
#5110=ORIENTED_EDGE('',*,*,#3769,.F.);
#5111=ORIENTED_EDGE('',*,*,#3809,.T.);
#5112=ORIENTED_EDGE('',*,*,#3644,.T.);
#5113=ORIENTED_EDGE('',*,*,#3809,.F.);
#5114=ORIENTED_EDGE('',*,*,#3768,.F.);
#5115=ORIENTED_EDGE('',*,*,#3810,.F.);
#5116=ORIENTED_EDGE('',*,*,#3645,.F.);
#5117=ORIENTED_EDGE('',*,*,#3810,.T.);
#5118=ORIENTED_EDGE('',*,*,#3767,.F.);
#5119=ORIENTED_EDGE('',*,*,#3811,.T.);
#5120=ORIENTED_EDGE('',*,*,#3646,.T.);
#5121=ORIENTED_EDGE('',*,*,#3811,.F.);
#5122=ORIENTED_EDGE('',*,*,#3766,.F.);
#5123=ORIENTED_EDGE('',*,*,#3812,.F.);
#5124=ORIENTED_EDGE('',*,*,#3647,.F.);
#5125=ORIENTED_EDGE('',*,*,#3812,.T.);
#5126=ORIENTED_EDGE('',*,*,#3765,.F.);
#5127=ORIENTED_EDGE('',*,*,#3813,.T.);
#5128=ORIENTED_EDGE('',*,*,#3648,.T.);
#5129=ORIENTED_EDGE('',*,*,#3813,.F.);
#5130=ORIENTED_EDGE('',*,*,#3764,.F.);
#5131=ORIENTED_EDGE('',*,*,#3814,.F.);
#5132=ORIENTED_EDGE('',*,*,#3649,.F.);
#5133=ORIENTED_EDGE('',*,*,#3814,.T.);
#5134=ORIENTED_EDGE('',*,*,#3763,.F.);
#5135=ORIENTED_EDGE('',*,*,#3815,.T.);
#5136=ORIENTED_EDGE('',*,*,#3650,.T.);
#5137=ORIENTED_EDGE('',*,*,#3815,.F.);
#5138=ORIENTED_EDGE('',*,*,#3762,.F.);
#5139=ORIENTED_EDGE('',*,*,#3816,.F.);
#5140=ORIENTED_EDGE('',*,*,#3651,.F.);
#5141=ORIENTED_EDGE('',*,*,#3816,.T.);
#5142=ORIENTED_EDGE('',*,*,#3761,.F.);
#5143=ORIENTED_EDGE('',*,*,#3817,.T.);
#5144=ORIENTED_EDGE('',*,*,#3652,.T.);
#5145=ORIENTED_EDGE('',*,*,#3817,.F.);
#5146=ORIENTED_EDGE('',*,*,#3760,.F.);
#5147=ORIENTED_EDGE('',*,*,#3818,.F.);
#5148=ORIENTED_EDGE('',*,*,#3653,.F.);
#5149=ORIENTED_EDGE('',*,*,#3818,.T.);
#5150=ORIENTED_EDGE('',*,*,#3759,.F.);
#5151=ORIENTED_EDGE('',*,*,#3819,.T.);
#5152=ORIENTED_EDGE('',*,*,#3654,.T.);
#5153=ORIENTED_EDGE('',*,*,#3819,.F.);
#5154=ORIENTED_EDGE('',*,*,#3758,.F.);
#5155=ORIENTED_EDGE('',*,*,#3820,.F.);
#5156=ORIENTED_EDGE('',*,*,#3655,.F.);
#5157=ORIENTED_EDGE('',*,*,#3820,.T.);
#5158=ORIENTED_EDGE('',*,*,#3757,.F.);
#5159=ORIENTED_EDGE('',*,*,#3821,.T.);
#5160=ORIENTED_EDGE('',*,*,#3656,.T.);
#5161=ORIENTED_EDGE('',*,*,#3821,.F.);
#5162=ORIENTED_EDGE('',*,*,#3756,.F.);
#5163=ORIENTED_EDGE('',*,*,#3822,.F.);
#5164=ORIENTED_EDGE('',*,*,#3657,.F.);
#5165=ORIENTED_EDGE('',*,*,#3822,.T.);
#5166=ORIENTED_EDGE('',*,*,#3755,.F.);
#5167=ORIENTED_EDGE('',*,*,#3823,.T.);
#5168=ORIENTED_EDGE('',*,*,#3658,.T.);
#5169=ORIENTED_EDGE('',*,*,#3823,.F.);
#5170=ORIENTED_EDGE('',*,*,#3754,.F.);
#5171=ORIENTED_EDGE('',*,*,#3824,.F.);
#5172=ORIENTED_EDGE('',*,*,#3659,.F.);
#5173=ORIENTED_EDGE('',*,*,#3824,.T.);
#5174=ORIENTED_EDGE('',*,*,#3753,.F.);
#5175=ORIENTED_EDGE('',*,*,#3825,.T.);
#5176=ORIENTED_EDGE('',*,*,#3660,.T.);
#5177=ORIENTED_EDGE('',*,*,#3825,.F.);
#5178=ORIENTED_EDGE('',*,*,#3752,.F.);
#5179=ORIENTED_EDGE('',*,*,#3826,.F.);
#5180=ORIENTED_EDGE('',*,*,#3661,.F.);
#5181=ORIENTED_EDGE('',*,*,#3826,.T.);
#5182=ORIENTED_EDGE('',*,*,#3751,.F.);
#5183=ORIENTED_EDGE('',*,*,#3827,.T.);
#5184=ORIENTED_EDGE('',*,*,#3662,.T.);
#5185=ORIENTED_EDGE('',*,*,#3827,.F.);
#5186=ORIENTED_EDGE('',*,*,#3750,.F.);
#5187=ORIENTED_EDGE('',*,*,#3828,.F.);
#5188=ORIENTED_EDGE('',*,*,#3663,.F.);
#5189=ORIENTED_EDGE('',*,*,#3828,.T.);
#5190=ORIENTED_EDGE('',*,*,#3749,.F.);
#5191=ORIENTED_EDGE('',*,*,#3829,.T.);
#5192=ORIENTED_EDGE('',*,*,#3664,.T.);
#5193=ORIENTED_EDGE('',*,*,#3829,.F.);
#5194=ORIENTED_EDGE('',*,*,#3748,.F.);
#5195=ORIENTED_EDGE('',*,*,#3830,.F.);
#5196=ORIENTED_EDGE('',*,*,#3665,.F.);
#5197=ORIENTED_EDGE('',*,*,#3830,.T.);
#5198=ORIENTED_EDGE('',*,*,#3747,.F.);
#5199=ORIENTED_EDGE('',*,*,#3831,.T.);
#5200=ORIENTED_EDGE('',*,*,#3666,.T.);
#5201=ORIENTED_EDGE('',*,*,#3831,.F.);
#5202=ORIENTED_EDGE('',*,*,#3746,.F.);
#5203=ORIENTED_EDGE('',*,*,#3832,.F.);
#5204=ORIENTED_EDGE('',*,*,#3667,.F.);
#5205=ORIENTED_EDGE('',*,*,#3832,.T.);
#5206=ORIENTED_EDGE('',*,*,#3745,.F.);
#5207=ORIENTED_EDGE('',*,*,#3833,.T.);
#5208=ORIENTED_EDGE('',*,*,#3668,.T.);
#5209=ORIENTED_EDGE('',*,*,#3833,.F.);
#5210=ORIENTED_EDGE('',*,*,#3744,.F.);
#5211=ORIENTED_EDGE('',*,*,#3834,.F.);
#5212=ORIENTED_EDGE('',*,*,#3669,.F.);
#5213=ORIENTED_EDGE('',*,*,#3834,.T.);
#5214=ORIENTED_EDGE('',*,*,#3743,.F.);
#5215=ORIENTED_EDGE('',*,*,#3835,.T.);
#5216=ORIENTED_EDGE('',*,*,#3670,.T.);
#5217=ORIENTED_EDGE('',*,*,#3835,.F.);
#5218=ORIENTED_EDGE('',*,*,#3742,.F.);
#5219=ORIENTED_EDGE('',*,*,#3836,.F.);
#5220=ORIENTED_EDGE('',*,*,#3671,.F.);
#5221=ORIENTED_EDGE('',*,*,#3836,.T.);
#5222=ORIENTED_EDGE('',*,*,#3741,.F.);
#5223=ORIENTED_EDGE('',*,*,#3837,.T.);
#5224=ORIENTED_EDGE('',*,*,#3672,.T.);
#5225=ORIENTED_EDGE('',*,*,#3837,.F.);
#5226=ORIENTED_EDGE('',*,*,#3740,.F.);
#5227=ORIENTED_EDGE('',*,*,#3838,.F.);
#5228=ORIENTED_EDGE('',*,*,#3673,.F.);
#5229=ORIENTED_EDGE('',*,*,#3838,.T.);
#5230=ORIENTED_EDGE('',*,*,#3739,.F.);
#5231=ORIENTED_EDGE('',*,*,#3839,.T.);
#5232=ORIENTED_EDGE('',*,*,#3674,.T.);
#5233=ORIENTED_EDGE('',*,*,#3839,.F.);
#5234=ORIENTED_EDGE('',*,*,#3738,.F.);
#5235=ORIENTED_EDGE('',*,*,#3840,.F.);
#5236=ORIENTED_EDGE('',*,*,#3675,.F.);
#5237=ORIENTED_EDGE('',*,*,#3840,.T.);
#5238=ORIENTED_EDGE('',*,*,#3737,.F.);
#5239=ORIENTED_EDGE('',*,*,#3841,.T.);
#5240=ORIENTED_EDGE('',*,*,#3676,.T.);
#5241=ORIENTED_EDGE('',*,*,#3841,.F.);
#5242=ORIENTED_EDGE('',*,*,#3736,.F.);
#5243=ORIENTED_EDGE('',*,*,#3842,.F.);
#5244=ORIENTED_EDGE('',*,*,#3677,.F.);
#5245=ORIENTED_EDGE('',*,*,#3842,.T.);
#5246=ORIENTED_EDGE('',*,*,#3735,.F.);
#5247=ORIENTED_EDGE('',*,*,#3843,.T.);
#5248=ORIENTED_EDGE('',*,*,#3678,.T.);
#5249=ORIENTED_EDGE('',*,*,#3843,.F.);
#5250=ORIENTED_EDGE('',*,*,#3734,.F.);
#5251=ORIENTED_EDGE('',*,*,#3844,.F.);
#5252=ORIENTED_EDGE('',*,*,#3679,.F.);
#5253=ORIENTED_EDGE('',*,*,#3844,.T.);
#5254=ORIENTED_EDGE('',*,*,#3733,.F.);
#5255=ORIENTED_EDGE('',*,*,#3845,.T.);
#5256=ORIENTED_EDGE('',*,*,#3680,.T.);
#5257=ORIENTED_EDGE('',*,*,#3845,.F.);
#5258=ORIENTED_EDGE('',*,*,#3732,.F.);
#5259=ORIENTED_EDGE('',*,*,#3846,.F.);
#5260=ORIENTED_EDGE('',*,*,#3681,.F.);
#5261=ORIENTED_EDGE('',*,*,#3846,.T.);
#5262=ORIENTED_EDGE('',*,*,#3731,.F.);
#5263=ORIENTED_EDGE('',*,*,#3847,.T.);
#5264=ORIENTED_EDGE('',*,*,#3682,.T.);
#5265=ORIENTED_EDGE('',*,*,#3847,.F.);
#5266=ORIENTED_EDGE('',*,*,#3730,.F.);
#5267=ORIENTED_EDGE('',*,*,#3848,.F.);
#5268=ORIENTED_EDGE('',*,*,#3683,.F.);
#5269=ORIENTED_EDGE('',*,*,#3848,.T.);
#5270=ORIENTED_EDGE('',*,*,#3729,.F.);
#5271=ORIENTED_EDGE('',*,*,#3849,.T.);
#5272=ORIENTED_EDGE('',*,*,#3684,.T.);
#5273=ORIENTED_EDGE('',*,*,#3849,.F.);
#5274=ORIENTED_EDGE('',*,*,#3728,.F.);
#5275=ORIENTED_EDGE('',*,*,#3850,.F.);
#5276=ORIENTED_EDGE('',*,*,#3685,.F.);
#5277=ORIENTED_EDGE('',*,*,#3850,.T.);
#5278=ORIENTED_EDGE('',*,*,#3727,.F.);
#5279=ORIENTED_EDGE('',*,*,#3851,.T.);
#5280=ORIENTED_EDGE('',*,*,#3686,.T.);
#5281=ORIENTED_EDGE('',*,*,#3851,.F.);
#5282=ORIENTED_EDGE('',*,*,#3726,.F.);
#5283=ORIENTED_EDGE('',*,*,#3852,.F.);
#5284=ORIENTED_EDGE('',*,*,#3687,.F.);
#5285=ORIENTED_EDGE('',*,*,#3852,.T.);
#5286=ORIENTED_EDGE('',*,*,#3725,.F.);
#5287=ORIENTED_EDGE('',*,*,#3853,.T.);
#5288=ORIENTED_EDGE('',*,*,#3688,.T.);
#5289=ORIENTED_EDGE('',*,*,#3853,.F.);
#5290=ORIENTED_EDGE('',*,*,#3724,.F.);
#5291=ORIENTED_EDGE('',*,*,#3854,.F.);
#5292=ORIENTED_EDGE('',*,*,#3689,.F.);
#5293=ORIENTED_EDGE('',*,*,#3854,.T.);
#5294=ORIENTED_EDGE('',*,*,#3723,.F.);
#5295=ORIENTED_EDGE('',*,*,#3855,.T.);
#5296=ORIENTED_EDGE('',*,*,#3690,.T.);
#5297=ORIENTED_EDGE('',*,*,#3855,.F.);
#5298=ORIENTED_EDGE('',*,*,#3722,.F.);
#5299=ORIENTED_EDGE('',*,*,#3856,.F.);
#5300=ORIENTED_EDGE('',*,*,#3691,.F.);
#5301=ORIENTED_EDGE('',*,*,#3856,.T.);
#5302=ORIENTED_EDGE('',*,*,#3721,.F.);
#5303=ORIENTED_EDGE('',*,*,#3857,.T.);
#5304=ORIENTED_EDGE('',*,*,#3692,.T.);
#5305=ORIENTED_EDGE('',*,*,#3857,.F.);
#5306=ORIENTED_EDGE('',*,*,#3720,.F.);
#5307=ORIENTED_EDGE('',*,*,#3858,.F.);
#5308=ORIENTED_EDGE('',*,*,#3693,.F.);
#5309=ORIENTED_EDGE('',*,*,#3858,.T.);
#5310=ORIENTED_EDGE('',*,*,#3719,.F.);
#5311=ORIENTED_EDGE('',*,*,#3859,.T.);
#5312=ORIENTED_EDGE('',*,*,#3694,.T.);
#5313=ORIENTED_EDGE('',*,*,#3859,.F.);
#5314=ORIENTED_EDGE('',*,*,#3718,.F.);
#5315=ORIENTED_EDGE('',*,*,#3860,.F.);
#5316=ORIENTED_EDGE('',*,*,#3695,.F.);
#5317=ORIENTED_EDGE('',*,*,#3860,.T.);
#5318=ORIENTED_EDGE('',*,*,#3717,.F.);
#5319=ORIENTED_EDGE('',*,*,#3861,.T.);
#5320=ORIENTED_EDGE('',*,*,#3696,.T.);
#5321=ORIENTED_EDGE('',*,*,#3861,.F.);
#5322=ORIENTED_EDGE('',*,*,#3716,.F.);
#5323=ORIENTED_EDGE('',*,*,#3862,.F.);
#5324=ORIENTED_EDGE('',*,*,#3697,.F.);
#5325=ORIENTED_EDGE('',*,*,#3862,.T.);
#5326=ORIENTED_EDGE('',*,*,#3715,.F.);
#5327=ORIENTED_EDGE('',*,*,#3863,.T.);
#5328=ORIENTED_EDGE('',*,*,#3698,.T.);
#5329=ORIENTED_EDGE('',*,*,#3863,.F.);
#5330=ORIENTED_EDGE('',*,*,#3714,.F.);
#5331=ORIENTED_EDGE('',*,*,#3864,.F.);
#5332=ORIENTED_EDGE('',*,*,#3699,.F.);
#5333=ORIENTED_EDGE('',*,*,#3864,.T.);
#5334=ORIENTED_EDGE('',*,*,#3713,.F.);
#5335=ORIENTED_EDGE('',*,*,#3865,.T.);
#5336=ORIENTED_EDGE('',*,*,#3700,.T.);
#5337=ORIENTED_EDGE('',*,*,#3866,.F.);
#5338=ORIENTED_EDGE('',*,*,#3701,.F.);
#5339=ORIENTED_EDGE('',*,*,#3865,.F.);
#5340=ORIENTED_EDGE('',*,*,#3712,.F.);
#5341=ORIENTED_EDGE('',*,*,#3789,.T.);
#5342=ORIENTED_EDGE('',*,*,#3704,.T.);
#5343=ORIENTED_EDGE('',*,*,#3867,.T.);
#5344=ORIENTED_EDGE('',*,*,#3709,.F.);
#5345=ORIENTED_EDGE('',*,*,#3868,.F.);
#5346=ORIENTED_EDGE('',*,*,#3710,.F.);
#5347=ORIENTED_EDGE('',*,*,#3867,.F.);
#5348=ORIENTED_EDGE('',*,*,#3703,.F.);
#5349=ORIENTED_EDGE('',*,*,#3866,.T.);
#5350=ORIENTED_EDGE('',*,*,#3711,.F.);
#5351=ORIENTED_EDGE('',*,*,#3868,.T.);
#5352=ORIENTED_EDGE('',*,*,#3702,.T.);
#5691=CYLINDRICAL_SURFACE('',#6815,0.6);
#5692=CYLINDRICAL_SURFACE('',#6817,0.125);
#5693=CYLINDRICAL_SURFACE('',#6818,0.125);
#5694=CYLINDRICAL_SURFACE('',#6819,1.);
#5695=CYLINDRICAL_SURFACE('',#6822,0.125);
#5696=CYLINDRICAL_SURFACE('',#6823,0.125);
#5697=CYLINDRICAL_SURFACE('',#6907,1.4);
#5698=CYLINDRICAL_SURFACE('',#6992,1.4);
#5699=CYLINDRICAL_SURFACE('',#6993,0.0555000000000001);
#5700=CYLINDRICAL_SURFACE('',#6994,1.24783954473516);
#5701=CYLINDRICAL_SURFACE('',#6995,0.0555000000000001);
#5702=CYLINDRICAL_SURFACE('',#6996,1.24783954473516);
#5703=CYLINDRICAL_SURFACE('',#6997,0.0555000000000001);
#5704=CYLINDRICAL_SURFACE('',#6998,1.24783954473516);
#5705=CYLINDRICAL_SURFACE('',#6999,0.0555000000000001);
#5706=CYLINDRICAL_SURFACE('',#7000,1.24783954473516);
#5707=CYLINDRICAL_SURFACE('',#7001,0.0555000000000001);
#5708=CYLINDRICAL_SURFACE('',#7002,1.24783954473516);
#5709=CYLINDRICAL_SURFACE('',#7003,0.0555000000000001);
#5710=CYLINDRICAL_SURFACE('',#7004,1.24783954473516);
#5711=CYLINDRICAL_SURFACE('',#7005,0.0555000000000001);
#5712=CYLINDRICAL_SURFACE('',#7006,1.24783954473516);
#5713=CYLINDRICAL_SURFACE('',#7007,0.0555000000000001);
#5714=CYLINDRICAL_SURFACE('',#7008,1.24783954473516);
#5715=CYLINDRICAL_SURFACE('',#7009,0.0555000000000001);
#5716=CYLINDRICAL_SURFACE('',#7010,1.24783954473516);
#5717=CYLINDRICAL_SURFACE('',#7011,0.0555000000000001);
#5718=CYLINDRICAL_SURFACE('',#7012,1.24783954473516);
#5719=CYLINDRICAL_SURFACE('',#7013,0.0555000000000001);
#5720=CYLINDRICAL_SURFACE('',#7014,1.24783954473516);
#5721=CYLINDRICAL_SURFACE('',#7015,0.0555000000000001);
#5722=CYLINDRICAL_SURFACE('',#7016,1.24783954473516);
#5723=CYLINDRICAL_SURFACE('',#7017,0.0555000000000001);
#5724=CYLINDRICAL_SURFACE('',#7018,1.24783954473516);
#5725=CYLINDRICAL_SURFACE('',#7019,0.0555000000000001);
#5726=CYLINDRICAL_SURFACE('',#7020,1.24783954473516);
#5727=CYLINDRICAL_SURFACE('',#7021,0.0555000000000001);
#5728=CYLINDRICAL_SURFACE('',#7022,1.24783954473516);
#5729=CYLINDRICAL_SURFACE('',#7023,0.0555000000000001);
#5730=CYLINDRICAL_SURFACE('',#7024,1.24783954473516);
#5731=CYLINDRICAL_SURFACE('',#7025,0.0555000000000001);
#5732=CYLINDRICAL_SURFACE('',#7026,1.24783954473516);
#5733=CYLINDRICAL_SURFACE('',#7027,0.0555000000000001);
#5734=CYLINDRICAL_SURFACE('',#7028,1.24783954473516);
#5735=CYLINDRICAL_SURFACE('',#7029,0.0555000000000001);
#5736=CYLINDRICAL_SURFACE('',#7030,1.24783954473516);
#5737=CYLINDRICAL_SURFACE('',#7031,0.0555000000000001);
#5738=CYLINDRICAL_SURFACE('',#7032,1.24783954473516);
#5739=CYLINDRICAL_SURFACE('',#7033,0.0555000000000001);
#5740=CYLINDRICAL_SURFACE('',#7034,1.24783954473516);
#5741=CYLINDRICAL_SURFACE('',#7035,0.0555000000000001);
#5742=CYLINDRICAL_SURFACE('',#7036,1.24783954473516);
#5743=CYLINDRICAL_SURFACE('',#7037,0.0555000000000001);
#5744=CYLINDRICAL_SURFACE('',#7038,1.24783954473516);
#5745=CYLINDRICAL_SURFACE('',#7039,0.0555000000000001);
#5746=CYLINDRICAL_SURFACE('',#7040,1.24783954473516);
#5747=CYLINDRICAL_SURFACE('',#7041,0.0555000000000001);
#5748=CYLINDRICAL_SURFACE('',#7042,1.24783954473516);
#5749=CYLINDRICAL_SURFACE('',#7043,0.0555000000000001);
#5750=CYLINDRICAL_SURFACE('',#7044,1.24783954473516);
#5751=CYLINDRICAL_SURFACE('',#7045,0.0555000000000001);
#5752=CYLINDRICAL_SURFACE('',#7046,1.24783954473516);
#5753=CYLINDRICAL_SURFACE('',#7047,0.0555000000000001);
#5754=CYLINDRICAL_SURFACE('',#7048,1.24783954473516);
#5755=CYLINDRICAL_SURFACE('',#7049,0.0555000000000001);
#5756=CYLINDRICAL_SURFACE('',#7050,1.24783954473516);
#5757=CYLINDRICAL_SURFACE('',#7051,0.0555000000000001);
#5758=CYLINDRICAL_SURFACE('',#7052,1.24783954473516);
#5759=CYLINDRICAL_SURFACE('',#7053,0.0555000000000001);
#5760=CYLINDRICAL_SURFACE('',#7054,1.24783954473516);
#5761=CYLINDRICAL_SURFACE('',#7055,0.0555000000000001);
#5762=CYLINDRICAL_SURFACE('',#7056,1.24783954473516);
#5763=CYLINDRICAL_SURFACE('',#7057,0.0555000000000001);
#5764=CYLINDRICAL_SURFACE('',#7058,1.24783954473516);
#5765=CYLINDRICAL_SURFACE('',#7059,0.0555000000000001);
#5766=CYLINDRICAL_SURFACE('',#7060,1.24783954473516);
#5767=CYLINDRICAL_SURFACE('',#7061,0.0555000000000001);
#5768=CYLINDRICAL_SURFACE('',#7062,1.24783954473516);
#5769=CYLINDRICAL_SURFACE('',#7063,0.0555000000000001);
#5770=CYLINDRICAL_SURFACE('',#7064,1.24783954473516);
#5771=CYLINDRICAL_SURFACE('',#7065,0.0555000000000001);
#5772=CYLINDRICAL_SURFACE('',#7066,1.24783954473516);
#5773=CYLINDRICAL_SURFACE('',#7067,0.0555000000000001);
#5774=CYLINDRICAL_SURFACE('',#7068,1.24783954473516);
#5775=CYLINDRICAL_SURFACE('',#7069,0.0555000000000001);
#5776=CYLINDRICAL_SURFACE('',#7070,1.24783954473516);
#5777=CYLINDRICAL_SURFACE('',#7071,0.0555000000000001);
#5778=CYLINDRICAL_SURFACE('',#7072,1.24783954473516);
#5970=ADVANCED_FACE('',(#859),#616,.F.);
#5971=ADVANCED_FACE('',(#860,#488),#617,.F.);
#5972=ADVANCED_FACE('',(#861),#618,.F.);
#5973=ADVANCED_FACE('',(#862,#489),#619,.T.);
#5974=ADVANCED_FACE('',(#863,#490,#491,#492),#5691,.F.);
#5975=ADVANCED_FACE('',(#864),#5692,.F.);
#5976=ADVANCED_FACE('',(#865),#5693,.F.);
#5977=ADVANCED_FACE('',(#866,#493,#494,#495),#5694,.T.);
#5978=ADVANCED_FACE('',(#867),#5695,.F.);
#5979=ADVANCED_FACE('',(#868),#5696,.F.);
#5980=ADVANCED_FACE('',(#869,#496),#620,.F.);
#5981=ADVANCED_FACE('',(#870,#497),#621,.T.);
#5982=ADVANCED_FACE('',(#871),#5697,.T.);
#5983=ADVANCED_FACE('',(#872,#498),#622,.F.);
#5984=ADVANCED_FACE('',(#873,#499),#623,.F.);
#5985=ADVANCED_FACE('',(#874),#5698,.T.);
#5986=ADVANCED_FACE('',(#875),#5699,.F.);
#5987=ADVANCED_FACE('',(#876),#5700,.T.);
#5988=ADVANCED_FACE('',(#877),#5701,.F.);
#5989=ADVANCED_FACE('',(#878),#5702,.T.);
#5990=ADVANCED_FACE('',(#879),#5703,.F.);
#5991=ADVANCED_FACE('',(#880),#5704,.T.);
#5992=ADVANCED_FACE('',(#881),#5705,.F.);
#5993=ADVANCED_FACE('',(#882),#5706,.T.);
#5994=ADVANCED_FACE('',(#883),#5707,.F.);
#5995=ADVANCED_FACE('',(#884),#5708,.T.);
#5996=ADVANCED_FACE('',(#885),#5709,.F.);
#5997=ADVANCED_FACE('',(#886),#5710,.T.);
#5998=ADVANCED_FACE('',(#887),#5711,.F.);
#5999=ADVANCED_FACE('',(#888),#5712,.T.);
#6000=ADVANCED_FACE('',(#889),#5713,.F.);
#6001=ADVANCED_FACE('',(#890),#5714,.T.);
#6002=ADVANCED_FACE('',(#891),#5715,.F.);
#6003=ADVANCED_FACE('',(#892),#5716,.T.);
#6004=ADVANCED_FACE('',(#893),#5717,.F.);
#6005=ADVANCED_FACE('',(#894),#5718,.T.);
#6006=ADVANCED_FACE('',(#895),#5719,.F.);
#6007=ADVANCED_FACE('',(#896),#5720,.T.);
#6008=ADVANCED_FACE('',(#897),#5721,.F.);
#6009=ADVANCED_FACE('',(#898),#5722,.T.);
#6010=ADVANCED_FACE('',(#899),#5723,.F.);
#6011=ADVANCED_FACE('',(#900),#5724,.T.);
#6012=ADVANCED_FACE('',(#901),#5725,.F.);
#6013=ADVANCED_FACE('',(#902),#5726,.T.);
#6014=ADVANCED_FACE('',(#903),#5727,.F.);
#6015=ADVANCED_FACE('',(#904),#5728,.T.);
#6016=ADVANCED_FACE('',(#905),#5729,.F.);
#6017=ADVANCED_FACE('',(#906),#5730,.T.);
#6018=ADVANCED_FACE('',(#907),#5731,.F.);
#6019=ADVANCED_FACE('',(#908),#5732,.T.);
#6020=ADVANCED_FACE('',(#909),#5733,.F.);
#6021=ADVANCED_FACE('',(#910),#5734,.T.);
#6022=ADVANCED_FACE('',(#911),#5735,.F.);
#6023=ADVANCED_FACE('',(#912),#5736,.T.);
#6024=ADVANCED_FACE('',(#913),#5737,.F.);
#6025=ADVANCED_FACE('',(#914),#5738,.T.);
#6026=ADVANCED_FACE('',(#915),#5739,.F.);
#6027=ADVANCED_FACE('',(#916),#5740,.T.);
#6028=ADVANCED_FACE('',(#917),#5741,.F.);
#6029=ADVANCED_FACE('',(#918),#5742,.T.);
#6030=ADVANCED_FACE('',(#919),#5743,.F.);
#6031=ADVANCED_FACE('',(#920),#5744,.T.);
#6032=ADVANCED_FACE('',(#921),#5745,.F.);
#6033=ADVANCED_FACE('',(#922),#5746,.T.);
#6034=ADVANCED_FACE('',(#923),#5747,.F.);
#6035=ADVANCED_FACE('',(#924),#5748,.T.);
#6036=ADVANCED_FACE('',(#925),#5749,.F.);
#6037=ADVANCED_FACE('',(#926),#5750,.T.);
#6038=ADVANCED_FACE('',(#927),#5751,.F.);
#6039=ADVANCED_FACE('',(#928),#5752,.T.);
#6040=ADVANCED_FACE('',(#929),#5753,.F.);
#6041=ADVANCED_FACE('',(#930),#5754,.T.);
#6042=ADVANCED_FACE('',(#931),#5755,.F.);
#6043=ADVANCED_FACE('',(#932),#5756,.T.);
#6044=ADVANCED_FACE('',(#933),#5757,.F.);
#6045=ADVANCED_FACE('',(#934),#5758,.T.);
#6046=ADVANCED_FACE('',(#935),#5759,.F.);
#6047=ADVANCED_FACE('',(#936),#5760,.T.);
#6048=ADVANCED_FACE('',(#937),#5761,.F.);
#6049=ADVANCED_FACE('',(#938),#5762,.T.);
#6050=ADVANCED_FACE('',(#939),#5763,.F.);
#6051=ADVANCED_FACE('',(#940),#5764,.T.);
#6052=ADVANCED_FACE('',(#941),#5765,.F.);
#6053=ADVANCED_FACE('',(#942),#5766,.T.);
#6054=ADVANCED_FACE('',(#943),#5767,.F.);
#6055=ADVANCED_FACE('',(#944),#5768,.T.);
#6056=ADVANCED_FACE('',(#945),#5769,.F.);
#6057=ADVANCED_FACE('',(#946),#5770,.T.);
#6058=ADVANCED_FACE('',(#947),#5771,.F.);
#6059=ADVANCED_FACE('',(#948),#5772,.T.);
#6060=ADVANCED_FACE('',(#949),#5773,.F.);
#6061=ADVANCED_FACE('',(#950),#5774,.T.);
#6062=ADVANCED_FACE('',(#951),#5775,.F.);
#6063=ADVANCED_FACE('',(#952),#5776,.T.);
#6064=ADVANCED_FACE('',(#953),#5777,.F.);
#6065=ADVANCED_FACE('',(#954),#5778,.T.);
#6153=CLOSED_SHELL('',(#5970,#5971,#5972,#5973,#5974,#5975,#5976,#5977,
#5978,#5979,#5980,#5981,#5982,#5983,#5984,#5985,#5986,#5987,#5988,#5989,
#5990,#5991,#5992,#5993,#5994,#5995,#5996,#5997,#5998,#5999,#6000,#6001,
#6002,#6003,#6004,#6005,#6006,#6007,#6008,#6009,#6010,#6011,#6012,#6013,
#6014,#6015,#6016,#6017,#6018,#6019,#6020,#6021,#6022,#6023,#6024,#6025,
#6026,#6027,#6028,#6029,#6030,#6031,#6032,#6033,#6034,#6035,#6036,#6037,
#6038,#6039,#6040,#6041,#6042,#6043,#6044,#6045,#6046,#6047,#6048,#6049,
#6050,#6051,#6052,#6053,#6054,#6055,#6056,#6057,#6058,#6059,#6060,#6061,
#6062,#6063,#6064,#6065));
#6807=AXIS2_PLACEMENT_3D('',#10521,#8124,#8125);
#6808=AXIS2_PLACEMENT_3D('',#10522,#8126,#8127);
#6809=AXIS2_PLACEMENT_3D('',#10531,#8132,#8133);
#6810=AXIS2_PLACEMENT_3D('',#10538,#8137,#8138);
#6811=AXIS2_PLACEMENT_3D('',#10539,#8139,#8140);
#6812=AXIS2_PLACEMENT_3D('',#10545,#8144,#8145);
#6813=AXIS2_PLACEMENT_3D('',#10547,#8146,#8147);
#6814=AXIS2_PLACEMENT_3D('',#10548,#8148,#8149);
#6815=AXIS2_PLACEMENT_3D('',#10549,#8150,#8151);
#6816=AXIS2_PLACEMENT_3D('',#10550,#8152,#8153);
#6817=AXIS2_PLACEMENT_3D('',#10665,#8154,#8155);
#6818=AXIS2_PLACEMENT_3D('',#10708,#8157,#8158);
#6819=AXIS2_PLACEMENT_3D('',#10751,#8160,#8161);
#6820=AXIS2_PLACEMENT_3D('',#10753,#8162,#8163);
#6821=AXIS2_PLACEMENT_3D('',#10757,#8166,#8167);
#6822=AXIS2_PLACEMENT_3D('',#10840,#8168,#8169);
#6823=AXIS2_PLACEMENT_3D('',#10842,#8171,#8172);
#6824=AXIS2_PLACEMENT_3D('',#10844,#8174,#8175);
#6825=AXIS2_PLACEMENT_3D('',#10845,#8176,#8177);
#6826=AXIS2_PLACEMENT_3D('',#10847,#8178,#8179);
#6827=AXIS2_PLACEMENT_3D('',#10850,#8180,#8181);
#6828=AXIS2_PLACEMENT_3D('',#10852,#8182,#8183);
#6829=AXIS2_PLACEMENT_3D('',#10854,#8184,#8185);
#6830=AXIS2_PLACEMENT_3D('',#10856,#8186,#8187);
#6831=AXIS2_PLACEMENT_3D('',#10858,#8188,#8189);
#6832=AXIS2_PLACEMENT_3D('',#10860,#8190,#8191);
#6833=AXIS2_PLACEMENT_3D('',#10862,#8192,#8193);
#6834=AXIS2_PLACEMENT_3D('',#10864,#8194,#8195);
#6835=AXIS2_PLACEMENT_3D('',#10866,#8196,#8197);
#6836=AXIS2_PLACEMENT_3D('',#10868,#8198,#8199);
#6837=AXIS2_PLACEMENT_3D('',#10870,#8200,#8201);
#6838=AXIS2_PLACEMENT_3D('',#10872,#8202,#8203);
#6839=AXIS2_PLACEMENT_3D('',#10874,#8204,#8205);
#6840=AXIS2_PLACEMENT_3D('',#10876,#8206,#8207);
#6841=AXIS2_PLACEMENT_3D('',#10878,#8208,#8209);
#6842=AXIS2_PLACEMENT_3D('',#10880,#8210,#8211);
#6843=AXIS2_PLACEMENT_3D('',#10882,#8212,#8213);
#6844=AXIS2_PLACEMENT_3D('',#10884,#8214,#8215);
#6845=AXIS2_PLACEMENT_3D('',#10886,#8216,#8217);
#6846=AXIS2_PLACEMENT_3D('',#10888,#8218,#8219);
#6847=AXIS2_PLACEMENT_3D('',#10890,#8220,#8221);
#6848=AXIS2_PLACEMENT_3D('',#10892,#8222,#8223);
#6849=AXIS2_PLACEMENT_3D('',#10894,#8224,#8225);
#6850=AXIS2_PLACEMENT_3D('',#10896,#8226,#8227);
#6851=AXIS2_PLACEMENT_3D('',#10898,#8228,#8229);
#6852=AXIS2_PLACEMENT_3D('',#10900,#8230,#8231);
#6853=AXIS2_PLACEMENT_3D('',#10902,#8232,#8233);
#6854=AXIS2_PLACEMENT_3D('',#10904,#8234,#8235);
#6855=AXIS2_PLACEMENT_3D('',#10906,#8236,#8237);
#6856=AXIS2_PLACEMENT_3D('',#10908,#8238,#8239);
#6857=AXIS2_PLACEMENT_3D('',#10910,#8240,#8241);
#6858=AXIS2_PLACEMENT_3D('',#10912,#8242,#8243);
#6859=AXIS2_PLACEMENT_3D('',#10914,#8244,#8245);
#6860=AXIS2_PLACEMENT_3D('',#10916,#8246,#8247);
#6861=AXIS2_PLACEMENT_3D('',#10918,#8248,#8249);
#6862=AXIS2_PLACEMENT_3D('',#10920,#8250,#8251);
#6863=AXIS2_PLACEMENT_3D('',#10922,#8252,#8253);
#6864=AXIS2_PLACEMENT_3D('',#10924,#8254,#8255);
#6865=AXIS2_PLACEMENT_3D('',#10926,#8256,#8257);
#6866=AXIS2_PLACEMENT_3D('',#10928,#8258,#8259);
#6867=AXIS2_PLACEMENT_3D('',#10930,#8260,#8261);
#6868=AXIS2_PLACEMENT_3D('',#10932,#8262,#8263);
#6869=AXIS2_PLACEMENT_3D('',#10934,#8264,#8265);
#6870=AXIS2_PLACEMENT_3D('',#10936,#8266,#8267);
#6871=AXIS2_PLACEMENT_3D('',#10938,#8268,#8269);
#6872=AXIS2_PLACEMENT_3D('',#10940,#8270,#8271);
#6873=AXIS2_PLACEMENT_3D('',#10942,#8272,#8273);
#6874=AXIS2_PLACEMENT_3D('',#10944,#8274,#8275);
#6875=AXIS2_PLACEMENT_3D('',#10946,#8276,#8277);
#6876=AXIS2_PLACEMENT_3D('',#10948,#8278,#8279);
#6877=AXIS2_PLACEMENT_3D('',#10950,#8280,#8281);
#6878=AXIS2_PLACEMENT_3D('',#10952,#8282,#8283);
#6879=AXIS2_PLACEMENT_3D('',#10954,#8284,#8285);
#6880=AXIS2_PLACEMENT_3D('',#10956,#8286,#8287);
#6881=AXIS2_PLACEMENT_3D('',#10958,#8288,#8289);
#6882=AXIS2_PLACEMENT_3D('',#10960,#8290,#8291);
#6883=AXIS2_PLACEMENT_3D('',#10962,#8292,#8293);
#6884=AXIS2_PLACEMENT_3D('',#10964,#8294,#8295);
#6885=AXIS2_PLACEMENT_3D('',#10966,#8296,#8297);
#6886=AXIS2_PLACEMENT_3D('',#10968,#8298,#8299);
#6887=AXIS2_PLACEMENT_3D('',#10970,#8300,#8301);
#6888=AXIS2_PLACEMENT_3D('',#10972,#8302,#8303);
#6889=AXIS2_PLACEMENT_3D('',#10974,#8304,#8305);
#6890=AXIS2_PLACEMENT_3D('',#10976,#8306,#8307);
#6891=AXIS2_PLACEMENT_3D('',#10978,#8308,#8309);
#6892=AXIS2_PLACEMENT_3D('',#10980,#8310,#8311);
#6893=AXIS2_PLACEMENT_3D('',#10982,#8312,#8313);
#6894=AXIS2_PLACEMENT_3D('',#10984,#8314,#8315);
#6895=AXIS2_PLACEMENT_3D('',#10986,#8316,#8317);
#6896=AXIS2_PLACEMENT_3D('',#10988,#8318,#8319);
#6897=AXIS2_PLACEMENT_3D('',#10990,#8320,#8321);
#6898=AXIS2_PLACEMENT_3D('',#10992,#8322,#8323);
#6899=AXIS2_PLACEMENT_3D('',#10994,#8324,#8325);
#6900=AXIS2_PLACEMENT_3D('',#10996,#8326,#8327);
#6901=AXIS2_PLACEMENT_3D('',#10998,#8328,#8329);
#6902=AXIS2_PLACEMENT_3D('',#11000,#8330,#8331);
#6903=AXIS2_PLACEMENT_3D('',#11002,#8332,#8333);
#6904=AXIS2_PLACEMENT_3D('',#11004,#8334,#8335);
#6905=AXIS2_PLACEMENT_3D('',#11006,#8336,#8337);
#6906=AXIS2_PLACEMENT_3D('',#11007,#8338,#8339);
#6907=AXIS2_PLACEMENT_3D('',#11008,#8340,#8341);
#6908=AXIS2_PLACEMENT_3D('',#11010,#8342,#8343);
#6909=AXIS2_PLACEMENT_3D('',#11012,#8345,#8346);
#6910=AXIS2_PLACEMENT_3D('',#11013,#8347,#8348);
#6911=AXIS2_PLACEMENT_3D('',#11015,#8349,#8350);
#6912=AXIS2_PLACEMENT_3D('',#11018,#8351,#8352);
#6913=AXIS2_PLACEMENT_3D('',#11020,#8353,#8354);
#6914=AXIS2_PLACEMENT_3D('',#11022,#8355,#8356);
#6915=AXIS2_PLACEMENT_3D('',#11024,#8357,#8358);
#6916=AXIS2_PLACEMENT_3D('',#11026,#8359,#8360);
#6917=AXIS2_PLACEMENT_3D('',#11028,#8361,#8362);
#6918=AXIS2_PLACEMENT_3D('',#11030,#8363,#8364);
#6919=AXIS2_PLACEMENT_3D('',#11032,#8365,#8366);
#6920=AXIS2_PLACEMENT_3D('',#11034,#8367,#8368);
#6921=AXIS2_PLACEMENT_3D('',#11036,#8369,#8370);
#6922=AXIS2_PLACEMENT_3D('',#11038,#8371,#8372);
#6923=AXIS2_PLACEMENT_3D('',#11040,#8373,#8374);
#6924=AXIS2_PLACEMENT_3D('',#11042,#8375,#8376);
#6925=AXIS2_PLACEMENT_3D('',#11044,#8377,#8378);
#6926=AXIS2_PLACEMENT_3D('',#11046,#8379,#8380);
#6927=AXIS2_PLACEMENT_3D('',#11048,#8381,#8382);
#6928=AXIS2_PLACEMENT_3D('',#11050,#8383,#8384);
#6929=AXIS2_PLACEMENT_3D('',#11052,#8385,#8386);
#6930=AXIS2_PLACEMENT_3D('',#11054,#8387,#8388);
#6931=AXIS2_PLACEMENT_3D('',#11056,#8389,#8390);
#6932=AXIS2_PLACEMENT_3D('',#11058,#8391,#8392);
#6933=AXIS2_PLACEMENT_3D('',#11060,#8393,#8394);
#6934=AXIS2_PLACEMENT_3D('',#11062,#8395,#8396);
#6935=AXIS2_PLACEMENT_3D('',#11064,#8397,#8398);
#6936=AXIS2_PLACEMENT_3D('',#11066,#8399,#8400);
#6937=AXIS2_PLACEMENT_3D('',#11068,#8401,#8402);
#6938=AXIS2_PLACEMENT_3D('',#11070,#8403,#8404);
#6939=AXIS2_PLACEMENT_3D('',#11072,#8405,#8406);
#6940=AXIS2_PLACEMENT_3D('',#11074,#8407,#8408);
#6941=AXIS2_PLACEMENT_3D('',#11076,#8409,#8410);
#6942=AXIS2_PLACEMENT_3D('',#11078,#8411,#8412);
#6943=AXIS2_PLACEMENT_3D('',#11080,#8413,#8414);
#6944=AXIS2_PLACEMENT_3D('',#11082,#8415,#8416);
#6945=AXIS2_PLACEMENT_3D('',#11084,#8417,#8418);
#6946=AXIS2_PLACEMENT_3D('',#11086,#8419,#8420);
#6947=AXIS2_PLACEMENT_3D('',#11088,#8421,#8422);
#6948=AXIS2_PLACEMENT_3D('',#11090,#8423,#8424);
#6949=AXIS2_PLACEMENT_3D('',#11092,#8425,#8426);
#6950=AXIS2_PLACEMENT_3D('',#11094,#8427,#8428);
#6951=AXIS2_PLACEMENT_3D('',#11096,#8429,#8430);
#6952=AXIS2_PLACEMENT_3D('',#11098,#8431,#8432);
#6953=AXIS2_PLACEMENT_3D('',#11100,#8433,#8434);
#6954=AXIS2_PLACEMENT_3D('',#11102,#8435,#8436);
#6955=AXIS2_PLACEMENT_3D('',#11104,#8437,#8438);
#6956=AXIS2_PLACEMENT_3D('',#11106,#8439,#8440);
#6957=AXIS2_PLACEMENT_3D('',#11108,#8441,#8442);
#6958=AXIS2_PLACEMENT_3D('',#11110,#8443,#8444);
#6959=AXIS2_PLACEMENT_3D('',#11112,#8445,#8446);
#6960=AXIS2_PLACEMENT_3D('',#11114,#8447,#8448);
#6961=AXIS2_PLACEMENT_3D('',#11116,#8449,#8450);
#6962=AXIS2_PLACEMENT_3D('',#11118,#8451,#8452);
#6963=AXIS2_PLACEMENT_3D('',#11120,#8453,#8454);
#6964=AXIS2_PLACEMENT_3D('',#11122,#8455,#8456);
#6965=AXIS2_PLACEMENT_3D('',#11124,#8457,#8458);
#6966=AXIS2_PLACEMENT_3D('',#11126,#8459,#8460);
#6967=AXIS2_PLACEMENT_3D('',#11128,#8461,#8462);
#6968=AXIS2_PLACEMENT_3D('',#11130,#8463,#8464);
#6969=AXIS2_PLACEMENT_3D('',#11132,#8465,#8466);
#6970=AXIS2_PLACEMENT_3D('',#11134,#8467,#8468);
#6971=AXIS2_PLACEMENT_3D('',#11136,#8469,#8470);
#6972=AXIS2_PLACEMENT_3D('',#11138,#8471,#8472);
#6973=AXIS2_PLACEMENT_3D('',#11140,#8473,#8474);
#6974=AXIS2_PLACEMENT_3D('',#11142,#8475,#8476);
#6975=AXIS2_PLACEMENT_3D('',#11144,#8477,#8478);
#6976=AXIS2_PLACEMENT_3D('',#11146,#8479,#8480);
#6977=AXIS2_PLACEMENT_3D('',#11148,#8481,#8482);
#6978=AXIS2_PLACEMENT_3D('',#11150,#8483,#8484);
#6979=AXIS2_PLACEMENT_3D('',#11152,#8485,#8486);
#6980=AXIS2_PLACEMENT_3D('',#11154,#8487,#8488);
#6981=AXIS2_PLACEMENT_3D('',#11156,#8489,#8490);
#6982=AXIS2_PLACEMENT_3D('',#11158,#8491,#8492);
#6983=AXIS2_PLACEMENT_3D('',#11160,#8493,#8494);
#6984=AXIS2_PLACEMENT_3D('',#11162,#8495,#8496);
#6985=AXIS2_PLACEMENT_3D('',#11164,#8497,#8498);
#6986=AXIS2_PLACEMENT_3D('',#11166,#8499,#8500);
#6987=AXIS2_PLACEMENT_3D('',#11168,#8501,#8502);
#6988=AXIS2_PLACEMENT_3D('',#11170,#8503,#8504);
#6989=AXIS2_PLACEMENT_3D('',#11172,#8505,#8506);
#6990=AXIS2_PLACEMENT_3D('',#11174,#8507,#8508);
#6991=AXIS2_PLACEMENT_3D('',#11175,#8509,#8510);
#6992=AXIS2_PLACEMENT_3D('',#11176,#8511,#8512);
#6993=AXIS2_PLACEMENT_3D('',#11178,#8514,#8515);
#6994=AXIS2_PLACEMENT_3D('',#11181,#8518,#8519);
#6995=AXIS2_PLACEMENT_3D('',#11183,#8521,#8522);
#6996=AXIS2_PLACEMENT_3D('',#11185,#8524,#8525);
#6997=AXIS2_PLACEMENT_3D('',#11187,#8527,#8528);
#6998=AXIS2_PLACEMENT_3D('',#11189,#8530,#8531);
#6999=AXIS2_PLACEMENT_3D('',#11191,#8533,#8534);
#7000=AXIS2_PLACEMENT_3D('',#11193,#8536,#8537);
#7001=AXIS2_PLACEMENT_3D('',#11195,#8539,#8540);
#7002=AXIS2_PLACEMENT_3D('',#11197,#8542,#8543);
#7003=AXIS2_PLACEMENT_3D('',#11199,#8545,#8546);
#7004=AXIS2_PLACEMENT_3D('',#11201,#8548,#8549);
#7005=AXIS2_PLACEMENT_3D('',#11203,#8551,#8552);
#7006=AXIS2_PLACEMENT_3D('',#11205,#8554,#8555);
#7007=AXIS2_PLACEMENT_3D('',#11207,#8557,#8558);
#7008=AXIS2_PLACEMENT_3D('',#11209,#8560,#8561);
#7009=AXIS2_PLACEMENT_3D('',#11211,#8563,#8564);
#7010=AXIS2_PLACEMENT_3D('',#11213,#8566,#8567);
#7011=AXIS2_PLACEMENT_3D('',#11215,#8569,#8570);
#7012=AXIS2_PLACEMENT_3D('',#11217,#8572,#8573);
#7013=AXIS2_PLACEMENT_3D('',#11219,#8575,#8576);
#7014=AXIS2_PLACEMENT_3D('',#11221,#8578,#8579);
#7015=AXIS2_PLACEMENT_3D('',#11223,#8581,#8582);
#7016=AXIS2_PLACEMENT_3D('',#11225,#8584,#8585);
#7017=AXIS2_PLACEMENT_3D('',#11227,#8587,#8588);
#7018=AXIS2_PLACEMENT_3D('',#11229,#8590,#8591);
#7019=AXIS2_PLACEMENT_3D('',#11231,#8593,#8594);
#7020=AXIS2_PLACEMENT_3D('',#11233,#8596,#8597);
#7021=AXIS2_PLACEMENT_3D('',#11235,#8599,#8600);
#7022=AXIS2_PLACEMENT_3D('',#11237,#8602,#8603);
#7023=AXIS2_PLACEMENT_3D('',#11239,#8605,#8606);
#7024=AXIS2_PLACEMENT_3D('',#11241,#8608,#8609);
#7025=AXIS2_PLACEMENT_3D('',#11243,#8611,#8612);
#7026=AXIS2_PLACEMENT_3D('',#11245,#8614,#8615);
#7027=AXIS2_PLACEMENT_3D('',#11247,#8617,#8618);
#7028=AXIS2_PLACEMENT_3D('',#11249,#8620,#8621);
#7029=AXIS2_PLACEMENT_3D('',#11251,#8623,#8624);
#7030=AXIS2_PLACEMENT_3D('',#11253,#8626,#8627);
#7031=AXIS2_PLACEMENT_3D('',#11255,#8629,#8630);
#7032=AXIS2_PLACEMENT_3D('',#11257,#8632,#8633);
#7033=AXIS2_PLACEMENT_3D('',#11259,#8635,#8636);
#7034=AXIS2_PLACEMENT_3D('',#11261,#8638,#8639);
#7035=AXIS2_PLACEMENT_3D('',#11263,#8641,#8642);
#7036=AXIS2_PLACEMENT_3D('',#11265,#8644,#8645);
#7037=AXIS2_PLACEMENT_3D('',#11267,#8647,#8648);
#7038=AXIS2_PLACEMENT_3D('',#11269,#8650,#8651);
#7039=AXIS2_PLACEMENT_3D('',#11271,#8653,#8654);
#7040=AXIS2_PLACEMENT_3D('',#11273,#8656,#8657);
#7041=AXIS2_PLACEMENT_3D('',#11275,#8659,#8660);
#7042=AXIS2_PLACEMENT_3D('',#11277,#8662,#8663);
#7043=AXIS2_PLACEMENT_3D('',#11279,#8665,#8666);
#7044=AXIS2_PLACEMENT_3D('',#11281,#8668,#8669);
#7045=AXIS2_PLACEMENT_3D('',#11283,#8671,#8672);
#7046=AXIS2_PLACEMENT_3D('',#11285,#8674,#8675);
#7047=AXIS2_PLACEMENT_3D('',#11287,#8677,#8678);
#7048=AXIS2_PLACEMENT_3D('',#11289,#8680,#8681);
#7049=AXIS2_PLACEMENT_3D('',#11291,#8683,#8684);
#7050=AXIS2_PLACEMENT_3D('',#11293,#8686,#8687);
#7051=AXIS2_PLACEMENT_3D('',#11295,#8689,#8690);
#7052=AXIS2_PLACEMENT_3D('',#11297,#8692,#8693);
#7053=AXIS2_PLACEMENT_3D('',#11299,#8695,#8696);
#7054=AXIS2_PLACEMENT_3D('',#11301,#8698,#8699);
#7055=AXIS2_PLACEMENT_3D('',#11303,#8701,#8702);
#7056=AXIS2_PLACEMENT_3D('',#11305,#8704,#8705);
#7057=AXIS2_PLACEMENT_3D('',#11307,#8707,#8708);
#7058=AXIS2_PLACEMENT_3D('',#11309,#8710,#8711);
#7059=AXIS2_PLACEMENT_3D('',#11311,#8713,#8714);
#7060=AXIS2_PLACEMENT_3D('',#11313,#8716,#8717);
#7061=AXIS2_PLACEMENT_3D('',#11315,#8719,#8720);
#7062=AXIS2_PLACEMENT_3D('',#11317,#8722,#8723);
#7063=AXIS2_PLACEMENT_3D('',#11319,#8725,#8726);
#7064=AXIS2_PLACEMENT_3D('',#11321,#8728,#8729);
#7065=AXIS2_PLACEMENT_3D('',#11323,#8731,#8732);
#7066=AXIS2_PLACEMENT_3D('',#11325,#8734,#8735);
#7067=AXIS2_PLACEMENT_3D('',#11327,#8737,#8738);
#7068=AXIS2_PLACEMENT_3D('',#11329,#8740,#8741);
#7069=AXIS2_PLACEMENT_3D('',#11331,#8743,#8744);
#7070=AXIS2_PLACEMENT_3D('',#11333,#8746,#8747);
#7071=AXIS2_PLACEMENT_3D('',#11335,#8749,#8750);
#7072=AXIS2_PLACEMENT_3D('',#11337,#8752,#8753);
#8124=DIRECTION('axis',(0.,0.,1.));
#8125=DIRECTION('refdir',(1.,0.,0.));
#8126=DIRECTION('center_axis',(-1.,0.,0.));
#8127=DIRECTION('ref_axis',(0.,0.,1.));
#8128=DIRECTION('',(0.,0.,1.));
#8129=DIRECTION('',(0.,1.,0.));
#8130=DIRECTION('',(0.,0.,-1.));
#8131=DIRECTION('',(0.,1.,0.));
#8132=DIRECTION('center_axis',(0.,0.,-1.));
#8133=DIRECTION('ref_axis',(-1.,0.,0.));
#8134=DIRECTION('',(-1.,0.,0.));
#8135=DIRECTION('',(0.,1.,0.));
#8136=DIRECTION('',(1.,0.,0.));
#8137=DIRECTION('center_axis',(0.,0.,1.));
#8138=DIRECTION('ref_axis',(1.,0.,0.));
#8139=DIRECTION('center_axis',(1.,0.,0.));
#8140=DIRECTION('ref_axis',(0.,0.,-1.));
#8141=DIRECTION('',(0.,0.,-1.));
#8142=DIRECTION('',(0.,-1.,0.));
#8143=DIRECTION('',(0.,0.,1.));
#8144=DIRECTION('center_axis',(0.,1.,0.));
#8145=DIRECTION('ref_axis',(1.,0.,0.));
#8146=DIRECTION('center_axis',(0.,1.,0.));
#8147=DIRECTION('ref_axis',(1.,0.,0.));
#8148=DIRECTION('center_axis',(0.,-1.,0.));
#8149=DIRECTION('ref_axis',(1.,0.,0.));
#8150=DIRECTION('center_axis',(0.,1.,0.));
#8151=DIRECTION('ref_axis',(-1.83697019872103E-16,0.,1.));
#8152=DIRECTION('center_axis',(0.,1.,0.));
#8153=DIRECTION('ref_axis',(1.,0.,0.));
#8154=DIRECTION('center_axis',(1.,0.,6.12323399573677E-17));
#8155=DIRECTION('ref_axis',(6.12323399573677E-17,0.,-1.));
#8156=DIRECTION('',(1.,0.,6.12323399573677E-17));
#8157=DIRECTION('center_axis',(1.,0.,6.12323399573677E-17));
#8158=DIRECTION('ref_axis',(6.12323399573677E-17,0.,-1.));
#8159=DIRECTION('',(1.,0.,6.12323399573677E-17));
#8160=DIRECTION('center_axis',(0.,-1.,0.));
#8161=DIRECTION('ref_axis',(1.,0.,0.));
#8162=DIRECTION('center_axis',(0.,-1.,0.));
#8163=DIRECTION('ref_axis',(1.,0.,0.));
#8164=DIRECTION('',(0.,1.,0.));
#8165=DIRECTION('',(0.,1.,0.));
#8166=DIRECTION('center_axis',(0.,1.,0.));
#8167=DIRECTION('ref_axis',(1.,0.,0.));
#8168=DIRECTION('center_axis',(0.,0.,1.));
#8169=DIRECTION('ref_axis',(1.,0.,0.));
#8170=DIRECTION('',(0.,0.,1.));
#8171=DIRECTION('center_axis',(0.,0.,1.));
#8172=DIRECTION('ref_axis',(1.,0.,0.));
#8173=DIRECTION('',(0.,0.,1.));
#8174=DIRECTION('center_axis',(0.,1.,0.));
#8175=DIRECTION('ref_axis',(1.,0.,0.));
#8176=DIRECTION('center_axis',(0.,1.,0.));
#8177=DIRECTION('ref_axis',(1.,0.,0.));
#8178=DIRECTION('center_axis',(0.,1.,0.));
#8179=DIRECTION('ref_axis',(1.,0.,0.));
#8180=DIRECTION('center_axis',(0.,1.,0.));
#8181=DIRECTION('ref_axis',(0.987688340595138,0.,0.156434465040231));
#8182=DIRECTION('center_axis',(0.,1.,0.));
#8183=DIRECTION('ref_axis',(1.,0.,0.));
#8184=DIRECTION('center_axis',(0.,1.,0.));
#8185=DIRECTION('ref_axis',(0.951056516295154,0.,0.309016994374948));
#8186=DIRECTION('center_axis',(0.,1.,0.));
#8187=DIRECTION('ref_axis',(1.,0.,0.));
#8188=DIRECTION('center_axis',(0.,1.,0.));
#8189=DIRECTION('ref_axis',(0.891006524188368,0.,0.453990499739547));
#8190=DIRECTION('center_axis',(0.,1.,0.));
#8191=DIRECTION('ref_axis',(1.,0.,0.));
#8192=DIRECTION('center_axis',(0.,1.,0.));
#8193=DIRECTION('ref_axis',(0.809016994374947,0.,0.587785252292473));
#8194=DIRECTION('center_axis',(0.,1.,0.));
#8195=DIRECTION('ref_axis',(1.,0.,0.));
#8196=DIRECTION('center_axis',(0.,1.,0.));
#8197=DIRECTION('ref_axis',(0.707106781186547,0.,0.707106781186548));
#8198=DIRECTION('center_axis',(0.,1.,0.));
#8199=DIRECTION('ref_axis',(1.,0.,0.));
#8200=DIRECTION('center_axis',(0.,1.,0.));
#8201=DIRECTION('ref_axis',(0.587785252292473,0.,0.809016994374948));
#8202=DIRECTION('center_axis',(0.,1.,0.));
#8203=DIRECTION('ref_axis',(1.,0.,0.));
#8204=DIRECTION('center_axis',(0.,1.,0.));
#8205=DIRECTION('ref_axis',(0.453990499739547,0.,0.891006524188368));
#8206=DIRECTION('center_axis',(0.,1.,0.));
#8207=DIRECTION('ref_axis',(1.,0.,0.));
#8208=DIRECTION('center_axis',(0.,1.,0.));
#8209=DIRECTION('ref_axis',(0.309016994374947,0.,0.951056516295154));
#8210=DIRECTION('center_axis',(0.,1.,0.));
#8211=DIRECTION('ref_axis',(1.,0.,0.));
#8212=DIRECTION('center_axis',(0.,1.,0.));
#8213=DIRECTION('ref_axis',(0.156434465040231,0.,0.987688340595138));
#8214=DIRECTION('center_axis',(0.,1.,0.));
#8215=DIRECTION('ref_axis',(1.,0.,0.));
#8216=DIRECTION('center_axis',(0.,1.,0.));
#8217=DIRECTION('ref_axis',(-1.83697019872103E-16,0.,1.));
#8218=DIRECTION('center_axis',(0.,1.,0.));
#8219=DIRECTION('ref_axis',(1.,0.,0.));
#8220=DIRECTION('center_axis',(0.,1.,0.));
#8221=DIRECTION('ref_axis',(-0.156434465040231,0.,0.987688340595138));
#8222=DIRECTION('center_axis',(0.,1.,0.));
#8223=DIRECTION('ref_axis',(1.,0.,0.));
#8224=DIRECTION('center_axis',(0.,1.,0.));
#8225=DIRECTION('ref_axis',(-0.309016994374948,0.,0.951056516295154));
#8226=DIRECTION('center_axis',(0.,1.,0.));
#8227=DIRECTION('ref_axis',(1.,0.,0.));
#8228=DIRECTION('center_axis',(0.,1.,0.));
#8229=DIRECTION('ref_axis',(-0.453990499739547,0.,0.891006524188368));
#8230=DIRECTION('center_axis',(0.,1.,0.));
#8231=DIRECTION('ref_axis',(1.,0.,0.));
#8232=DIRECTION('center_axis',(0.,1.,0.));
#8233=DIRECTION('ref_axis',(-0.587785252292473,0.,0.809016994374947));
#8234=DIRECTION('center_axis',(0.,1.,0.));
#8235=DIRECTION('ref_axis',(1.,0.,0.));
#8236=DIRECTION('center_axis',(0.,1.,0.));
#8237=DIRECTION('ref_axis',(-0.707106781186548,0.,0.707106781186547));
#8238=DIRECTION('center_axis',(0.,1.,0.));
#8239=DIRECTION('ref_axis',(1.,0.,0.));
#8240=DIRECTION('center_axis',(0.,1.,0.));
#8241=DIRECTION('ref_axis',(-0.809016994374947,0.,0.587785252292473));
#8242=DIRECTION('center_axis',(0.,1.,0.));
#8243=DIRECTION('ref_axis',(1.,0.,0.));
#8244=DIRECTION('center_axis',(0.,1.,0.));
#8245=DIRECTION('ref_axis',(-0.891006524188368,0.,0.453990499739547));
#8246=DIRECTION('center_axis',(0.,1.,0.));
#8247=DIRECTION('ref_axis',(1.,0.,0.));
#8248=DIRECTION('center_axis',(0.,1.,0.));
#8249=DIRECTION('ref_axis',(-0.951056516295154,0.,0.309016994374947));
#8250=DIRECTION('center_axis',(0.,1.,0.));
#8251=DIRECTION('ref_axis',(1.,0.,0.));
#8252=DIRECTION('center_axis',(0.,1.,0.));
#8253=DIRECTION('ref_axis',(-0.987688340595138,0.,0.156434465040231));
#8254=DIRECTION('center_axis',(0.,1.,0.));
#8255=DIRECTION('ref_axis',(1.,0.,0.));
#8256=DIRECTION('center_axis',(0.,1.,0.));
#8257=DIRECTION('ref_axis',(-1.,0.,-1.22464679914735E-16));
#8258=DIRECTION('center_axis',(0.,1.,0.));
#8259=DIRECTION('ref_axis',(1.,0.,0.));
#8260=DIRECTION('center_axis',(0.,1.,0.));
#8261=DIRECTION('ref_axis',(-0.987688340595138,0.,-0.156434465040231));
#8262=DIRECTION('center_axis',(0.,1.,0.));
#8263=DIRECTION('ref_axis',(1.,0.,0.));
#8264=DIRECTION('center_axis',(0.,1.,0.));
#8265=DIRECTION('ref_axis',(-0.951056516295154,0.,-0.309016994374948));
#8266=DIRECTION('center_axis',(0.,1.,0.));
#8267=DIRECTION('ref_axis',(1.,0.,0.));
#8268=DIRECTION('center_axis',(0.,1.,0.));
#8269=DIRECTION('ref_axis',(-0.891006524188368,0.,-0.453990499739547));
#8270=DIRECTION('center_axis',(0.,1.,0.));
#8271=DIRECTION('ref_axis',(1.,0.,0.));
#8272=DIRECTION('center_axis',(0.,1.,0.));
#8273=DIRECTION('ref_axis',(-0.809016994374947,0.,-0.587785252292473));
#8274=DIRECTION('center_axis',(0.,1.,0.));
#8275=DIRECTION('ref_axis',(1.,0.,0.));
#8276=DIRECTION('center_axis',(0.,1.,0.));
#8277=DIRECTION('ref_axis',(-0.707106781186547,0.,-0.707106781186548));
#8278=DIRECTION('center_axis',(0.,1.,0.));
#8279=DIRECTION('ref_axis',(1.,0.,0.));
#8280=DIRECTION('center_axis',(0.,1.,0.));
#8281=DIRECTION('ref_axis',(-0.587785252292473,0.,-0.809016994374947));
#8282=DIRECTION('center_axis',(0.,1.,0.));
#8283=DIRECTION('ref_axis',(1.,0.,0.));
#8284=DIRECTION('center_axis',(0.,1.,0.));
#8285=DIRECTION('ref_axis',(-0.453990499739547,0.,-0.891006524188368));
#8286=DIRECTION('center_axis',(0.,1.,0.));
#8287=DIRECTION('ref_axis',(1.,0.,0.));
#8288=DIRECTION('center_axis',(0.,1.,0.));
#8289=DIRECTION('ref_axis',(-0.309016994374947,0.,-0.951056516295154));
#8290=DIRECTION('center_axis',(0.,1.,0.));
#8291=DIRECTION('ref_axis',(1.,0.,0.));
#8292=DIRECTION('center_axis',(0.,1.,0.));
#8293=DIRECTION('ref_axis',(-0.156434465040231,0.,-0.987688340595138));
#8294=DIRECTION('center_axis',(0.,1.,0.));
#8295=DIRECTION('ref_axis',(1.,0.,0.));
#8296=DIRECTION('center_axis',(0.,1.,0.));
#8297=DIRECTION('ref_axis',(6.12323399573677E-17,0.,-1.));
#8298=DIRECTION('center_axis',(0.,1.,0.));
#8299=DIRECTION('ref_axis',(1.,0.,0.));
#8300=DIRECTION('center_axis',(0.,1.,0.));
#8301=DIRECTION('ref_axis',(0.156434465040231,0.,-0.987688340595138));
#8302=DIRECTION('center_axis',(0.,1.,0.));
#8303=DIRECTION('ref_axis',(1.,0.,0.));
#8304=DIRECTION('center_axis',(0.,1.,0.));
#8305=DIRECTION('ref_axis',(0.309016994374948,0.,-0.951056516295154));
#8306=DIRECTION('center_axis',(0.,1.,0.));
#8307=DIRECTION('ref_axis',(1.,0.,0.));
#8308=DIRECTION('center_axis',(0.,1.,0.));
#8309=DIRECTION('ref_axis',(0.453990499739547,0.,-0.891006524188368));
#8310=DIRECTION('center_axis',(0.,1.,0.));
#8311=DIRECTION('ref_axis',(1.,0.,0.));
#8312=DIRECTION('center_axis',(0.,1.,0.));
#8313=DIRECTION('ref_axis',(0.587785252292473,0.,-0.809016994374947));
#8314=DIRECTION('center_axis',(0.,1.,0.));
#8315=DIRECTION('ref_axis',(1.,0.,0.));
#8316=DIRECTION('center_axis',(0.,1.,0.));
#8317=DIRECTION('ref_axis',(0.707106781186548,0.,-0.707106781186547));
#8318=DIRECTION('center_axis',(0.,1.,0.));
#8319=DIRECTION('ref_axis',(1.,0.,0.));
#8320=DIRECTION('center_axis',(0.,1.,0.));
#8321=DIRECTION('ref_axis',(0.809016994374947,0.,-0.587785252292473));
#8322=DIRECTION('center_axis',(0.,1.,0.));
#8323=DIRECTION('ref_axis',(1.,0.,0.));
#8324=DIRECTION('center_axis',(0.,1.,0.));
#8325=DIRECTION('ref_axis',(0.891006524188368,0.,-0.453990499739547));
#8326=DIRECTION('center_axis',(0.,1.,0.));
#8327=DIRECTION('ref_axis',(1.,0.,0.));
#8328=DIRECTION('center_axis',(0.,1.,0.));
#8329=DIRECTION('ref_axis',(0.951056516295154,0.,-0.309016994374947));
#8330=DIRECTION('center_axis',(0.,1.,0.));
#8331=DIRECTION('ref_axis',(1.,0.,0.));
#8332=DIRECTION('center_axis',(0.,1.,0.));
#8333=DIRECTION('ref_axis',(0.987688340595138,0.,-0.156434465040231));
#8334=DIRECTION('center_axis',(0.,1.,0.));
#8335=DIRECTION('ref_axis',(1.,0.,0.));
#8336=DIRECTION('center_axis',(0.,1.,0.));
#8337=DIRECTION('ref_axis',(1.,0.,0.));
#8338=DIRECTION('center_axis',(0.,1.,0.));
#8339=DIRECTION('ref_axis',(1.,0.,0.));
#8340=DIRECTION('center_axis',(0.,-1.,0.));
#8341=DIRECTION('ref_axis',(1.,0.,0.));
#8342=DIRECTION('center_axis',(0.,-1.,0.));
#8343=DIRECTION('ref_axis',(1.,0.,0.));
#8344=DIRECTION('',(0.,1.,0.));
#8345=DIRECTION('center_axis',(0.,1.,0.));
#8346=DIRECTION('ref_axis',(1.,0.,0.));
#8347=DIRECTION('center_axis',(0.,1.,0.));
#8348=DIRECTION('ref_axis',(1.,0.,0.));
#8349=DIRECTION('center_axis',(0.,1.,0.));
#8350=DIRECTION('ref_axis',(1.,0.,0.));
#8351=DIRECTION('center_axis',(0.,-1.,0.));
#8352=DIRECTION('ref_axis',(0.987688340595138,0.,0.156434465040231));
#8353=DIRECTION('center_axis',(0.,1.,0.));
#8354=DIRECTION('ref_axis',(1.,0.,0.));
#8355=DIRECTION('center_axis',(0.,-1.,0.));
#8356=DIRECTION('ref_axis',(1.,0.,0.));
#8357=DIRECTION('center_axis',(0.,1.,0.));
#8358=DIRECTION('ref_axis',(1.,0.,0.));
#8359=DIRECTION('center_axis',(0.,-1.,0.));
#8360=DIRECTION('ref_axis',(0.987688340595138,0.,-0.156434465040231));
#8361=DIRECTION('center_axis',(0.,1.,0.));
#8362=DIRECTION('ref_axis',(1.,0.,0.));
#8363=DIRECTION('center_axis',(0.,-1.,0.));
#8364=DIRECTION('ref_axis',(0.951056516295154,0.,-0.309016994374947));
#8365=DIRECTION('center_axis',(0.,1.,0.));
#8366=DIRECTION('ref_axis',(1.,0.,0.));
#8367=DIRECTION('center_axis',(0.,-1.,0.));
#8368=DIRECTION('ref_axis',(0.891006524188368,0.,-0.453990499739547));
#8369=DIRECTION('center_axis',(0.,1.,0.));
#8370=DIRECTION('ref_axis',(1.,0.,0.));
#8371=DIRECTION('center_axis',(0.,-1.,0.));
#8372=DIRECTION('ref_axis',(0.809016994374947,0.,-0.587785252292473));
#8373=DIRECTION('center_axis',(0.,1.,0.));
#8374=DIRECTION('ref_axis',(1.,0.,0.));
#8375=DIRECTION('center_axis',(0.,-1.,0.));
#8376=DIRECTION('ref_axis',(0.707106781186548,0.,-0.707106781186547));
#8377=DIRECTION('center_axis',(0.,1.,0.));
#8378=DIRECTION('ref_axis',(1.,0.,0.));
#8379=DIRECTION('center_axis',(0.,-1.,0.));
#8380=DIRECTION('ref_axis',(0.587785252292473,0.,-0.809016994374947));
#8381=DIRECTION('center_axis',(0.,1.,0.));
#8382=DIRECTION('ref_axis',(1.,0.,0.));
#8383=DIRECTION('center_axis',(0.,-1.,0.));
#8384=DIRECTION('ref_axis',(0.453990499739547,0.,-0.891006524188368));
#8385=DIRECTION('center_axis',(0.,1.,0.));
#8386=DIRECTION('ref_axis',(1.,0.,0.));
#8387=DIRECTION('center_axis',(0.,-1.,0.));
#8388=DIRECTION('ref_axis',(0.309016994374948,0.,-0.951056516295154));
#8389=DIRECTION('center_axis',(0.,1.,0.));
#8390=DIRECTION('ref_axis',(1.,0.,0.));
#8391=DIRECTION('center_axis',(0.,-1.,0.));
#8392=DIRECTION('ref_axis',(0.156434465040231,0.,-0.987688340595138));
#8393=DIRECTION('center_axis',(0.,1.,0.));
#8394=DIRECTION('ref_axis',(1.,0.,0.));
#8395=DIRECTION('center_axis',(0.,-1.,0.));
#8396=DIRECTION('ref_axis',(6.12323399573677E-17,0.,-1.));
#8397=DIRECTION('center_axis',(0.,1.,0.));
#8398=DIRECTION('ref_axis',(1.,0.,0.));
#8399=DIRECTION('center_axis',(0.,-1.,0.));
#8400=DIRECTION('ref_axis',(-0.156434465040231,0.,-0.987688340595138));
#8401=DIRECTION('center_axis',(0.,1.,0.));
#8402=DIRECTION('ref_axis',(1.,0.,0.));
#8403=DIRECTION('center_axis',(0.,-1.,0.));
#8404=DIRECTION('ref_axis',(-0.309016994374947,0.,-0.951056516295154));
#8405=DIRECTION('center_axis',(0.,1.,0.));
#8406=DIRECTION('ref_axis',(1.,0.,0.));
#8407=DIRECTION('center_axis',(0.,-1.,0.));
#8408=DIRECTION('ref_axis',(-0.453990499739547,0.,-0.891006524188368));
#8409=DIRECTION('center_axis',(0.,1.,0.));
#8410=DIRECTION('ref_axis',(1.,0.,0.));
#8411=DIRECTION('center_axis',(0.,-1.,0.));
#8412=DIRECTION('ref_axis',(-0.587785252292473,0.,-0.809016994374947));
#8413=DIRECTION('center_axis',(0.,1.,0.));
#8414=DIRECTION('ref_axis',(1.,0.,0.));
#8415=DIRECTION('center_axis',(0.,-1.,0.));
#8416=DIRECTION('ref_axis',(-0.707106781186547,0.,-0.707106781186548));
#8417=DIRECTION('center_axis',(0.,1.,0.));
#8418=DIRECTION('ref_axis',(1.,0.,0.));
#8419=DIRECTION('center_axis',(0.,-1.,0.));
#8420=DIRECTION('ref_axis',(-0.809016994374947,0.,-0.587785252292473));
#8421=DIRECTION('center_axis',(0.,1.,0.));
#8422=DIRECTION('ref_axis',(1.,0.,0.));
#8423=DIRECTION('center_axis',(0.,-1.,0.));
#8424=DIRECTION('ref_axis',(-0.891006524188368,0.,-0.453990499739547));
#8425=DIRECTION('center_axis',(0.,1.,0.));
#8426=DIRECTION('ref_axis',(1.,0.,0.));
#8427=DIRECTION('center_axis',(0.,-1.,0.));
#8428=DIRECTION('ref_axis',(-0.951056516295154,0.,-0.309016994374948));
#8429=DIRECTION('center_axis',(0.,1.,0.));
#8430=DIRECTION('ref_axis',(1.,0.,0.));
#8431=DIRECTION('center_axis',(0.,-1.,0.));
#8432=DIRECTION('ref_axis',(-0.987688340595138,0.,-0.156434465040231));
#8433=DIRECTION('center_axis',(0.,1.,0.));
#8434=DIRECTION('ref_axis',(1.,0.,0.));
#8435=DIRECTION('center_axis',(0.,-1.,0.));
#8436=DIRECTION('ref_axis',(-1.,0.,-1.22464679914735E-16));
#8437=DIRECTION('center_axis',(0.,1.,0.));
#8438=DIRECTION('ref_axis',(1.,0.,0.));
#8439=DIRECTION('center_axis',(0.,-1.,0.));
#8440=DIRECTION('ref_axis',(-0.987688340595138,0.,0.156434465040231));
#8441=DIRECTION('center_axis',(0.,1.,0.));
#8442=DIRECTION('ref_axis',(1.,0.,0.));
#8443=DIRECTION('center_axis',(0.,-1.,0.));
#8444=DIRECTION('ref_axis',(-0.951056516295154,0.,0.309016994374947));
#8445=DIRECTION('center_axis',(0.,1.,0.));
#8446=DIRECTION('ref_axis',(1.,0.,0.));
#8447=DIRECTION('center_axis',(0.,-1.,0.));
#8448=DIRECTION('ref_axis',(-0.891006524188368,0.,0.453990499739547));
#8449=DIRECTION('center_axis',(0.,1.,0.));
#8450=DIRECTION('ref_axis',(1.,0.,0.));
#8451=DIRECTION('center_axis',(0.,-1.,0.));
#8452=DIRECTION('ref_axis',(-0.809016994374947,0.,0.587785252292473));
#8453=DIRECTION('center_axis',(0.,1.,0.));
#8454=DIRECTION('ref_axis',(1.,0.,0.));
#8455=DIRECTION('center_axis',(0.,-1.,0.));
#8456=DIRECTION('ref_axis',(-0.707106781186548,0.,0.707106781186547));
#8457=DIRECTION('center_axis',(0.,1.,0.));
#8458=DIRECTION('ref_axis',(1.,0.,0.));
#8459=DIRECTION('center_axis',(0.,-1.,0.));
#8460=DIRECTION('ref_axis',(-0.587785252292473,0.,0.809016994374947));
#8461=DIRECTION('center_axis',(0.,1.,0.));
#8462=DIRECTION('ref_axis',(1.,0.,0.));
#8463=DIRECTION('center_axis',(0.,-1.,0.));
#8464=DIRECTION('ref_axis',(-0.453990499739547,0.,0.891006524188368));
#8465=DIRECTION('center_axis',(0.,1.,0.));
#8466=DIRECTION('ref_axis',(1.,0.,0.));
#8467=DIRECTION('center_axis',(0.,-1.,0.));
#8468=DIRECTION('ref_axis',(-0.309016994374948,0.,0.951056516295154));
#8469=DIRECTION('center_axis',(0.,1.,0.));
#8470=DIRECTION('ref_axis',(1.,0.,0.));
#8471=DIRECTION('center_axis',(0.,-1.,0.));
#8472=DIRECTION('ref_axis',(-0.156434465040231,0.,0.987688340595138));
#8473=DIRECTION('center_axis',(0.,1.,0.));
#8474=DIRECTION('ref_axis',(1.,0.,0.));
#8475=DIRECTION('center_axis',(0.,-1.,0.));
#8476=DIRECTION('ref_axis',(-1.83697019872103E-16,0.,1.));
#8477=DIRECTION('center_axis',(0.,1.,0.));
#8478=DIRECTION('ref_axis',(1.,0.,0.));
#8479=DIRECTION('center_axis',(0.,-1.,0.));
#8480=DIRECTION('ref_axis',(0.156434465040231,0.,0.987688340595138));
#8481=DIRECTION('center_axis',(0.,1.,0.));
#8482=DIRECTION('ref_axis',(1.,0.,0.));
#8483=DIRECTION('center_axis',(0.,-1.,0.));
#8484=DIRECTION('ref_axis',(0.309016994374947,0.,0.951056516295154));
#8485=DIRECTION('center_axis',(0.,1.,0.));
#8486=DIRECTION('ref_axis',(1.,0.,0.));
#8487=DIRECTION('center_axis',(0.,-1.,0.));
#8488=DIRECTION('ref_axis',(0.453990499739547,0.,0.891006524188368));
#8489=DIRECTION('center_axis',(0.,1.,0.));
#8490=DIRECTION('ref_axis',(1.,0.,0.));
#8491=DIRECTION('center_axis',(0.,-1.,0.));
#8492=DIRECTION('ref_axis',(0.587785252292473,0.,0.809016994374948));
#8493=DIRECTION('center_axis',(0.,1.,0.));
#8494=DIRECTION('ref_axis',(1.,0.,0.));
#8495=DIRECTION('center_axis',(0.,-1.,0.));
#8496=DIRECTION('ref_axis',(0.707106781186547,0.,0.707106781186548));
#8497=DIRECTION('center_axis',(0.,1.,0.));
#8498=DIRECTION('ref_axis',(1.,0.,0.));
#8499=DIRECTION('center_axis',(0.,-1.,0.));
#8500=DIRECTION('ref_axis',(0.809016994374947,0.,0.587785252292473));
#8501=DIRECTION('center_axis',(0.,1.,0.));
#8502=DIRECTION('ref_axis',(1.,0.,0.));
#8503=DIRECTION('center_axis',(0.,-1.,0.));
#8504=DIRECTION('ref_axis',(0.891006524188368,0.,0.453990499739547));
#8505=DIRECTION('center_axis',(0.,1.,0.));
#8506=DIRECTION('ref_axis',(1.,0.,0.));
#8507=DIRECTION('center_axis',(0.,-1.,0.));
#8508=DIRECTION('ref_axis',(0.951056516295154,0.,0.309016994374948));
#8509=DIRECTION('center_axis',(0.,1.,0.));
#8510=DIRECTION('ref_axis',(1.,0.,0.));
#8511=DIRECTION('center_axis',(0.,1.,0.));
#8512=DIRECTION('ref_axis',(1.,0.,0.));
#8513=DIRECTION('',(0.,-1.,0.));
#8514=DIRECTION('center_axis',(0.,1.,0.));
#8515=DIRECTION('ref_axis',(-0.987688340595137,0.,-0.156434465040233));
#8516=DIRECTION('',(0.,-1.,0.));
#8517=DIRECTION('',(0.,1.,0.));
#8518=DIRECTION('center_axis',(0.,1.,0.));
#8519=DIRECTION('ref_axis',(1.,0.,0.));
#8520=DIRECTION('',(0.,-1.,0.));
#8521=DIRECTION('center_axis',(0.,1.,0.));
#8522=DIRECTION('ref_axis',(-0.951056516295153,0.,-0.309016994374949));
#8523=DIRECTION('',(0.,1.,0.));
#8524=DIRECTION('center_axis',(0.,1.,0.));
#8525=DIRECTION('ref_axis',(1.,0.,0.));
#8526=DIRECTION('',(0.,-1.,0.));
#8527=DIRECTION('center_axis',(0.,1.,0.));
#8528=DIRECTION('ref_axis',(-0.891006524188368,0.,-0.453990499739547));
#8529=DIRECTION('',(0.,1.,0.));
#8530=DIRECTION('center_axis',(0.,1.,0.));
#8531=DIRECTION('ref_axis',(1.,0.,0.));
#8532=DIRECTION('',(0.,-1.,0.));
#8533=DIRECTION('center_axis',(0.,1.,0.));
#8534=DIRECTION('ref_axis',(-0.809016994374948,0.,-0.587785252292473));
#8535=DIRECTION('',(0.,1.,0.));
#8536=DIRECTION('center_axis',(0.,1.,0.));
#8537=DIRECTION('ref_axis',(1.,0.,0.));
#8538=DIRECTION('',(0.,-1.,0.));
#8539=DIRECTION('center_axis',(0.,1.,0.));
#8540=DIRECTION('ref_axis',(-0.707106781186547,0.,-0.707106781186548));
#8541=DIRECTION('',(0.,1.,0.));
#8542=DIRECTION('center_axis',(0.,1.,0.));
#8543=DIRECTION('ref_axis',(1.,0.,0.));
#8544=DIRECTION('',(0.,-1.,0.));
#8545=DIRECTION('center_axis',(0.,1.,0.));
#8546=DIRECTION('ref_axis',(-0.587785252292474,0.,-0.809016994374947));
#8547=DIRECTION('',(0.,1.,0.));
#8548=DIRECTION('center_axis',(0.,1.,0.));
#8549=DIRECTION('ref_axis',(1.,0.,0.));
#8550=DIRECTION('',(0.,-1.,0.));
#8551=DIRECTION('center_axis',(0.,1.,0.));
#8552=DIRECTION('ref_axis',(-0.453990499739547,0.,-0.891006524188368));
#8553=DIRECTION('',(0.,1.,0.));
#8554=DIRECTION('center_axis',(0.,1.,0.));
#8555=DIRECTION('ref_axis',(1.,0.,0.));
#8556=DIRECTION('',(0.,-1.,0.));
#8557=DIRECTION('center_axis',(0.,1.,0.));
#8558=DIRECTION('ref_axis',(-0.309016994374948,0.,-0.951056516295153));
#8559=DIRECTION('',(0.,1.,0.));
#8560=DIRECTION('center_axis',(0.,1.,0.));
#8561=DIRECTION('ref_axis',(1.,0.,0.));
#8562=DIRECTION('',(0.,-1.,0.));
#8563=DIRECTION('center_axis',(0.,1.,0.));
#8564=DIRECTION('ref_axis',(-0.156434465040232,0.,-0.987688340595138));
#8565=DIRECTION('',(0.,1.,0.));
#8566=DIRECTION('center_axis',(0.,1.,0.));
#8567=DIRECTION('ref_axis',(1.,0.,0.));
#8568=DIRECTION('',(0.,-1.,0.));
#8569=DIRECTION('center_axis',(0.,1.,0.));
#8570=DIRECTION('ref_axis',(3.06161699786838E-16,0.,-1.));
#8571=DIRECTION('',(0.,1.,0.));
#8572=DIRECTION('center_axis',(0.,1.,0.));
#8573=DIRECTION('ref_axis',(1.,0.,0.));
#8574=DIRECTION('',(0.,-1.,0.));
#8575=DIRECTION('center_axis',(0.,1.,0.));
#8576=DIRECTION('ref_axis',(0.156434465040233,0.,-0.987688340595138));
#8577=DIRECTION('',(0.,1.,0.));
#8578=DIRECTION('center_axis',(0.,1.,0.));
#8579=DIRECTION('ref_axis',(1.,0.,0.));
#8580=DIRECTION('',(0.,-1.,0.));
#8581=DIRECTION('center_axis',(0.,1.,0.));
#8582=DIRECTION('ref_axis',(0.309016994374946,0.,-0.951056516295154));
#8583=DIRECTION('',(0.,1.,0.));
#8584=DIRECTION('center_axis',(0.,1.,0.));
#8585=DIRECTION('ref_axis',(1.,0.,0.));
#8586=DIRECTION('',(0.,-1.,0.));
#8587=DIRECTION('center_axis',(0.,1.,0.));
#8588=DIRECTION('ref_axis',(0.453990499739547,0.,-0.891006524188368));
#8589=DIRECTION('',(0.,1.,0.));
#8590=DIRECTION('center_axis',(0.,1.,0.));
#8591=DIRECTION('ref_axis',(1.,0.,0.));
#8592=DIRECTION('',(0.,-1.,0.));
#8593=DIRECTION('center_axis',(0.,1.,0.));
#8594=DIRECTION('ref_axis',(0.587785252292473,0.,-0.809016994374947));
#8595=DIRECTION('',(0.,1.,0.));
#8596=DIRECTION('center_axis',(0.,1.,0.));
#8597=DIRECTION('ref_axis',(1.,0.,0.));
#8598=DIRECTION('',(0.,-1.,0.));
#8599=DIRECTION('center_axis',(0.,1.,0.));
#8600=DIRECTION('ref_axis',(0.707106781186548,0.,-0.707106781186547));
#8601=DIRECTION('',(0.,1.,0.));
#8602=DIRECTION('center_axis',(0.,1.,0.));
#8603=DIRECTION('ref_axis',(1.,0.,0.));
#8604=DIRECTION('',(0.,-1.,0.));
#8605=DIRECTION('center_axis',(0.,1.,0.));
#8606=DIRECTION('ref_axis',(0.809016994374946,0.,-0.587785252292475));
#8607=DIRECTION('',(0.,1.,0.));
#8608=DIRECTION('center_axis',(0.,1.,0.));
#8609=DIRECTION('ref_axis',(1.,0.,0.));
#8610=DIRECTION('',(0.,-1.,0.));
#8611=DIRECTION('center_axis',(0.,1.,0.));
#8612=DIRECTION('ref_axis',(0.891006524188368,0.,-0.453990499739547));
#8613=DIRECTION('',(0.,1.,0.));
#8614=DIRECTION('center_axis',(0.,1.,0.));
#8615=DIRECTION('ref_axis',(1.,0.,0.));
#8616=DIRECTION('',(0.,-1.,0.));
#8617=DIRECTION('center_axis',(0.,1.,0.));
#8618=DIRECTION('ref_axis',(0.951056516295154,0.,-0.309016994374946));
#8619=DIRECTION('',(0.,1.,0.));
#8620=DIRECTION('center_axis',(0.,1.,0.));
#8621=DIRECTION('ref_axis',(1.,0.,0.));
#8622=DIRECTION('',(0.,-1.,0.));
#8623=DIRECTION('center_axis',(0.,1.,0.));
#8624=DIRECTION('ref_axis',(0.987688340595138,0.,-0.156434465040232));
#8625=DIRECTION('',(0.,1.,0.));
#8626=DIRECTION('center_axis',(0.,1.,0.));
#8627=DIRECTION('ref_axis',(1.,0.,0.));
#8628=DIRECTION('',(0.,-1.,0.));
#8629=DIRECTION('center_axis',(0.,1.,0.));
#8630=DIRECTION('ref_axis',(1.,0.,2.44929359829471E-16));
#8631=DIRECTION('',(0.,1.,0.));
#8632=DIRECTION('center_axis',(0.,1.,0.));
#8633=DIRECTION('ref_axis',(1.,0.,0.));
#8634=DIRECTION('',(0.,-1.,0.));
#8635=DIRECTION('center_axis',(0.,1.,0.));
#8636=DIRECTION('ref_axis',(0.987688340595137,0.,0.156434465040232));
#8637=DIRECTION('',(0.,1.,0.));
#8638=DIRECTION('center_axis',(0.,1.,0.));
#8639=DIRECTION('ref_axis',(1.,0.,0.));
#8640=DIRECTION('',(0.,-1.,0.));
#8641=DIRECTION('center_axis',(0.,1.,0.));
#8642=DIRECTION('ref_axis',(0.951056516295154,0.,0.309016994374946));
#8643=DIRECTION('',(0.,1.,0.));
#8644=DIRECTION('center_axis',(0.,1.,0.));
#8645=DIRECTION('ref_axis',(1.,0.,0.));
#8646=DIRECTION('',(0.,-1.,0.));
#8647=DIRECTION('center_axis',(0.,1.,0.));
#8648=DIRECTION('ref_axis',(0.891006524188368,0.,0.453990499739547));
#8649=DIRECTION('',(0.,1.,0.));
#8650=DIRECTION('center_axis',(0.,1.,0.));
#8651=DIRECTION('ref_axis',(1.,0.,0.));
#8652=DIRECTION('',(0.,-1.,0.));
#8653=DIRECTION('center_axis',(0.,1.,0.));
#8654=DIRECTION('ref_axis',(0.809016994374947,0.,0.587785252292473));
#8655=DIRECTION('',(0.,1.,0.));
#8656=DIRECTION('center_axis',(0.,1.,0.));
#8657=DIRECTION('ref_axis',(1.,0.,0.));
#8658=DIRECTION('',(0.,-1.,0.));
#8659=DIRECTION('center_axis',(0.,1.,0.));
#8660=DIRECTION('ref_axis',(0.707106781186547,0.,0.707106781186548));
#8661=DIRECTION('',(0.,1.,0.));
#8662=DIRECTION('center_axis',(0.,1.,0.));
#8663=DIRECTION('ref_axis',(1.,0.,0.));
#8664=DIRECTION('',(0.,-1.,0.));
#8665=DIRECTION('center_axis',(0.,1.,0.));
#8666=DIRECTION('ref_axis',(0.587785252292475,0.,0.809016994374946));
#8667=DIRECTION('',(0.,1.,0.));
#8668=DIRECTION('center_axis',(0.,1.,0.));
#8669=DIRECTION('ref_axis',(1.,0.,0.));
#8670=DIRECTION('',(0.,-1.,0.));
#8671=DIRECTION('center_axis',(0.,1.,0.));
#8672=DIRECTION('ref_axis',(0.453990499739547,0.,0.891006524188368));
#8673=DIRECTION('',(0.,1.,0.));
#8674=DIRECTION('center_axis',(0.,1.,0.));
#8675=DIRECTION('ref_axis',(1.,0.,0.));
#8676=DIRECTION('',(0.,-1.,0.));
#8677=DIRECTION('center_axis',(0.,1.,0.));
#8678=DIRECTION('ref_axis',(0.309016994374946,0.,0.951056516295154));
#8679=DIRECTION('',(0.,1.,0.));
#8680=DIRECTION('center_axis',(0.,1.,0.));
#8681=DIRECTION('ref_axis',(1.,0.,0.));
#8682=DIRECTION('',(0.,-1.,0.));
#8683=DIRECTION('center_axis',(0.,1.,0.));
#8684=DIRECTION('ref_axis',(0.156434465040232,0.,0.987688340595138));
#8685=DIRECTION('',(0.,1.,0.));
#8686=DIRECTION('center_axis',(0.,1.,0.));
#8687=DIRECTION('ref_axis',(1.,0.,0.));
#8688=DIRECTION('',(0.,-1.,0.));
#8689=DIRECTION('center_axis',(0.,1.,0.));
#8690=DIRECTION('ref_axis',(-1.83697019872103E-16,0.,1.));
#8691=DIRECTION('',(0.,1.,0.));
#8692=DIRECTION('center_axis',(0.,1.,0.));
#8693=DIRECTION('ref_axis',(1.,0.,0.));
#8694=DIRECTION('',(0.,-1.,0.));
#8695=DIRECTION('center_axis',(0.,1.,0.));
#8696=DIRECTION('ref_axis',(-0.156434465040232,0.,0.987688340595138));
#8697=DIRECTION('',(0.,1.,0.));
#8698=DIRECTION('center_axis',(0.,1.,0.));
#8699=DIRECTION('ref_axis',(1.,0.,0.));
#8700=DIRECTION('',(0.,-1.,0.));
#8701=DIRECTION('center_axis',(0.,1.,0.));
#8702=DIRECTION('ref_axis',(-0.309016994374946,0.,0.951056516295154));
#8703=DIRECTION('',(0.,1.,0.));
#8704=DIRECTION('center_axis',(0.,1.,0.));
#8705=DIRECTION('ref_axis',(1.,0.,0.));
#8706=DIRECTION('',(0.,-1.,0.));
#8707=DIRECTION('center_axis',(0.,1.,0.));
#8708=DIRECTION('ref_axis',(-0.453990499739549,0.,0.891006524188367));
#8709=DIRECTION('',(0.,1.,0.));
#8710=DIRECTION('center_axis',(0.,1.,0.));
#8711=DIRECTION('ref_axis',(1.,0.,0.));
#8712=DIRECTION('',(0.,-1.,0.));
#8713=DIRECTION('center_axis',(0.,1.,0.));
#8714=DIRECTION('ref_axis',(-0.587785252292474,0.,0.809016994374947));
#8715=DIRECTION('',(0.,1.,0.));
#8716=DIRECTION('center_axis',(0.,1.,0.));
#8717=DIRECTION('ref_axis',(1.,0.,0.));
#8718=DIRECTION('',(0.,-1.,0.));
#8719=DIRECTION('center_axis',(0.,1.,0.));
#8720=DIRECTION('ref_axis',(-0.707106781186548,0.,0.707106781186547));
#8721=DIRECTION('',(0.,1.,0.));
#8722=DIRECTION('center_axis',(0.,1.,0.));
#8723=DIRECTION('ref_axis',(1.,0.,0.));
#8724=DIRECTION('',(0.,-1.,0.));
#8725=DIRECTION('center_axis',(0.,1.,0.));
#8726=DIRECTION('ref_axis',(-0.809016994374947,0.,0.587785252292474));
#8727=DIRECTION('',(0.,1.,0.));
#8728=DIRECTION('center_axis',(0.,1.,0.));
#8729=DIRECTION('ref_axis',(1.,0.,0.));
#8730=DIRECTION('',(0.,-1.,0.));
#8731=DIRECTION('center_axis',(0.,1.,0.));
#8732=DIRECTION('ref_axis',(-0.891006524188368,0.,0.453990499739547));
#8733=DIRECTION('',(0.,1.,0.));
#8734=DIRECTION('center_axis',(0.,1.,0.));
#8735=DIRECTION('ref_axis',(1.,0.,0.));
#8736=DIRECTION('',(0.,-1.,0.));
#8737=DIRECTION('center_axis',(0.,1.,0.));
#8738=DIRECTION('ref_axis',(-0.951056516295154,0.,0.309016994374948));
#8739=DIRECTION('',(0.,1.,0.));
#8740=DIRECTION('center_axis',(0.,1.,0.));
#8741=DIRECTION('ref_axis',(1.,0.,0.));
#8742=DIRECTION('',(0.,-1.,0.));
#8743=DIRECTION('center_axis',(0.,1.,0.));
#8744=DIRECTION('ref_axis',(-0.987688340595137,0.,0.156434465040233));
#8745=DIRECTION('',(0.,1.,0.));
#8746=DIRECTION('center_axis',(0.,1.,0.));
#8747=DIRECTION('ref_axis',(1.,0.,0.));
#8748=DIRECTION('',(0.,1.,0.));
#8749=DIRECTION('center_axis',(0.,1.,0.));
#8750=DIRECTION('ref_axis',(-1.,0.,-1.22464679914735E-16));
#8751=DIRECTION('',(0.,-1.,0.));
#8752=DIRECTION('center_axis',(0.,1.,0.));
#8753=DIRECTION('ref_axis',(1.,0.,0.));
#10521=CARTESIAN_POINT('',(0.,0.,0.));
#10522=CARTESIAN_POINT('Origin',(-0.2,-1.,-0.78));
#10523=CARTESIAN_POINT('',(-0.2,-0.9,-0.78));
#10524=CARTESIAN_POINT('',(-0.2,-0.9,-0.565685424949238));
#10525=CARTESIAN_POINT('',(-0.2,-0.9,-0.39));
#10526=CARTESIAN_POINT('',(-0.2,0.85,-0.78));
#10527=CARTESIAN_POINT('',(-0.2,-1.,-0.78));
#10528=CARTESIAN_POINT('',(-0.2,0.85,-0.565685424949238));
#10529=CARTESIAN_POINT('',(-0.2,0.85,-0.39));
#10530=CARTESIAN_POINT('',(-0.2,0.,-0.565685424949238));
#10531=CARTESIAN_POINT('Origin',(0.2,-1.,-0.78));
#10532=CARTESIAN_POINT('',(0.2,-0.9,-0.78));
#10533=CARTESIAN_POINT('',(0.1,-0.9,-0.78));
#10534=CARTESIAN_POINT('',(0.2,0.85,-0.78));
#10535=CARTESIAN_POINT('',(0.2,-1.,-0.78));
#10536=CARTESIAN_POINT('',(0.1,0.85,-0.78));
#10537=CARTESIAN_POINT('',(-0.125,-0.5,-0.78));
#10538=CARTESIAN_POINT('Origin',(0.,-0.5,-0.78));
#10539=CARTESIAN_POINT('Origin',(0.2,-1.,0.));
#10540=CARTESIAN_POINT('',(0.2,-0.9,-0.565685424949238));
#10541=CARTESIAN_POINT('',(0.2,-0.9,0.));
#10542=CARTESIAN_POINT('',(0.2,0.85,-0.565685424949238));
#10543=CARTESIAN_POINT('',(0.2,0.,-0.565685424949238));
#10544=CARTESIAN_POINT('',(0.2,0.85,0.));
#10545=CARTESIAN_POINT('Origin',(0.,0.85,0.));
#10546=CARTESIAN_POINT('',(-1.4,0.85,1.71450551880629E-16));
#10547=CARTESIAN_POINT('Origin',(0.,0.85,0.));
#10548=CARTESIAN_POINT('Origin',(0.,0.85,0.));
#10549=CARTESIAN_POINT('Origin',(0.,0.,0.));
#10550=CARTESIAN_POINT('Origin',(0.,-0.9,0.));
#10551=CARTESIAN_POINT('',(0.125,-0.5,0.586834729715275));
#10552=CARTESIAN_POINT('',(-0.125,-0.5,0.586834729715275));
#10553=CARTESIAN_POINT('Ctrl Pts',(0.125,-0.5,0.586834729715275));
#10554=CARTESIAN_POINT('Ctrl Pts',(0.125,-0.484254474936005,0.586834729715275));
#10555=CARTESIAN_POINT('Ctrl Pts',(0.121843784097853,-0.467492086231842,
0.587534197873268));
#10556=CARTESIAN_POINT('Ctrl Pts',(0.109073016834181,-0.436709004341607,
0.590038488226116));
#10557=CARTESIAN_POINT('Ctrl Pts',(0.0994608796208941,-0.422684184324257,
0.591804743154611));
#10558=CARTESIAN_POINT('Ctrl Pts',(0.077316548567853,-0.400539853271216,
0.59510289473619));
#10559=CARTESIAN_POINT('Ctrl Pts',(0.0632914182239686,-0.390927142361291,
0.596852269967858));
#10560=CARTESIAN_POINT('Ctrl Pts',(0.0325072544867634,-0.378155958502111,
0.599317707212167));
#10561=CARTESIAN_POINT('Ctrl Pts',(0.0157444828659572,-0.375,0.6));
#10562=CARTESIAN_POINT('Ctrl Pts',(-0.0157444828659573,-0.375,0.6));
#10563=CARTESIAN_POINT('Ctrl Pts',(-0.0325072544867634,-0.378155958502111,
0.599317707212167));
#10564=CARTESIAN_POINT('Ctrl Pts',(-0.0632914182239687,-0.390927142361291,
0.596852269967858));
#10565=CARTESIAN_POINT('Ctrl Pts',(-0.077316548567853,-0.400539853271216,
0.59510289473619));
#10566=CARTESIAN_POINT('Ctrl Pts',(-0.0994608796208942,-0.422684184324257,
0.591804743154611));
#10567=CARTESIAN_POINT('Ctrl Pts',(-0.109073016834181,-0.436709004341607,
0.590038488226116));
#10568=CARTESIAN_POINT('Ctrl Pts',(-0.121843784097853,-0.467492086231842,
0.587534197873268));
#10569=CARTESIAN_POINT('Ctrl Pts',(-0.125,-0.484254474936005,0.586834729715275));
#10570=CARTESIAN_POINT('Ctrl Pts',(-0.125,-0.5,0.586834729715275));
#10571=CARTESIAN_POINT('Ctrl Pts',(-0.125,-0.5,0.586834729715275));
#10572=CARTESIAN_POINT('Ctrl Pts',(-0.125,-0.515745525063995,0.586834729715275));
#10573=CARTESIAN_POINT('Ctrl Pts',(-0.121843784097853,-0.532507913768158,
0.587534197873268));
#10574=CARTESIAN_POINT('Ctrl Pts',(-0.109073016834181,-0.563290995658393,
0.590038488226116));
#10575=CARTESIAN_POINT('Ctrl Pts',(-0.0994608796208941,-0.577315815675743,
0.591804743154611));
#10576=CARTESIAN_POINT('Ctrl Pts',(-0.077316548567853,-0.599460146728784,
0.59510289473619));
#10577=CARTESIAN_POINT('Ctrl Pts',(-0.0632914182239687,-0.609072857638709,
0.596852269967858));
#10578=CARTESIAN_POINT('Ctrl Pts',(-0.0325072544867635,-0.621844041497889,
0.599317707212167));
#10579=CARTESIAN_POINT('Ctrl Pts',(-0.0157444828659572,-0.625,0.6));
#10580=CARTESIAN_POINT('Ctrl Pts',(0.0157444828659572,-0.625,0.6));
#10581=CARTESIAN_POINT('Ctrl Pts',(0.0325072544867633,-0.621844041497889,
0.599317707212167));
#10582=CARTESIAN_POINT('Ctrl Pts',(0.0632914182239686,-0.609072857638709,
0.596852269967858));
#10583=CARTESIAN_POINT('Ctrl Pts',(0.077316548567853,-0.599460146728784,
0.59510289473619));
#10584=CARTESIAN_POINT('Ctrl Pts',(0.0994608796208942,-0.577315815675743,
0.591804743154611));
#10585=CARTESIAN_POINT('Ctrl Pts',(0.109073016834181,-0.563290995658393,
0.590038488226116));
#10586=CARTESIAN_POINT('Ctrl Pts',(0.121843784097853,-0.532507913768158,
0.587534197873268));
#10587=CARTESIAN_POINT('Ctrl Pts',(0.125,-0.515745525063995,0.586834729715275));
#10588=CARTESIAN_POINT('Ctrl Pts',(0.125,-0.5,0.586834729715275));
#10589=CARTESIAN_POINT('',(-0.586834729715275,-0.5,-0.125));
#10590=CARTESIAN_POINT('',(-0.586834729715275,-0.5,0.125));
#10591=CARTESIAN_POINT('Ctrl Pts',(-0.586834729715275,-0.5,-0.125));
#10592=CARTESIAN_POINT('Ctrl Pts',(-0.586834729715275,-0.515745525063995,
-0.125));
#10593=CARTESIAN_POINT('Ctrl Pts',(-0.587534197873268,-0.532507913768158,
-0.121843784097853));
#10594=CARTESIAN_POINT('Ctrl Pts',(-0.590038488226116,-0.563290995658393,
-0.109073016834181));
#10595=CARTESIAN_POINT('Ctrl Pts',(-0.591804743154611,-0.577315815675743,
-0.0994608796208942));
#10596=CARTESIAN_POINT('Ctrl Pts',(-0.59510289473619,-0.599460146728784,
-0.0773165485678531));
#10597=CARTESIAN_POINT('Ctrl Pts',(-0.596852269967858,-0.609072857638709,
-0.0632914182239687));
#10598=CARTESIAN_POINT('Ctrl Pts',(-0.599317707212167,-0.621844041497889,
-0.0325072544867635));
#10599=CARTESIAN_POINT('Ctrl Pts',(-0.6,-0.625,-0.0157444828659573));
#10600=CARTESIAN_POINT('Ctrl Pts',(-0.6,-0.625,0.0157444828659572));
#10601=CARTESIAN_POINT('Ctrl Pts',(-0.599317707212167,-0.621844041497889,
0.0325072544867633));
#10602=CARTESIAN_POINT('Ctrl Pts',(-0.596852269967858,-0.609072857638709,
0.0632914182239686));
#10603=CARTESIAN_POINT('Ctrl Pts',(-0.59510289473619,-0.599460146728784,
0.077316548567853));
#10604=CARTESIAN_POINT('Ctrl Pts',(-0.591804743154611,-0.577315815675743,
0.0994608796208941));
#10605=CARTESIAN_POINT('Ctrl Pts',(-0.590038488226116,-0.563290995658393,
0.109073016834181));
#10606=CARTESIAN_POINT('Ctrl Pts',(-0.587534197873268,-0.532507913768158,
0.121843784097853));
#10607=CARTESIAN_POINT('Ctrl Pts',(-0.586834729715275,-0.515745525063995,
0.125));
#10608=CARTESIAN_POINT('Ctrl Pts',(-0.586834729715275,-0.5,0.125));
#10609=CARTESIAN_POINT('Ctrl Pts',(-0.586834729715275,-0.5,0.125));
#10610=CARTESIAN_POINT('Ctrl Pts',(-0.586834729715275,-0.484254474936005,
0.125));
#10611=CARTESIAN_POINT('Ctrl Pts',(-0.587534197873268,-0.467492086231842,
0.121843784097853));
#10612=CARTESIAN_POINT('Ctrl Pts',(-0.590038488226116,-0.436709004341607,
0.109073016834181));
#10613=CARTESIAN_POINT('Ctrl Pts',(-0.591804743154611,-0.422684184324257,
0.0994608796208941));
#10614=CARTESIAN_POINT('Ctrl Pts',(-0.59510289473619,-0.400539853271216,
0.077316548567853));
#10615=CARTESIAN_POINT('Ctrl Pts',(-0.596852269967858,-0.390927142361291,
0.0632914182239686));
#10616=CARTESIAN_POINT('Ctrl Pts',(-0.599317707212167,-0.378155958502111,
0.0325072544867634));
#10617=CARTESIAN_POINT('Ctrl Pts',(-0.6,-0.375,0.0157444828659572));
#10618=CARTESIAN_POINT('Ctrl Pts',(-0.6,-0.375,-0.0157444828659572));
#10619=CARTESIAN_POINT('Ctrl Pts',(-0.599317707212167,-0.378155958502111,
-0.0325072544867634));
#10620=CARTESIAN_POINT('Ctrl Pts',(-0.596852269967858,-0.390927142361291,
-0.0632914182239686));
#10621=CARTESIAN_POINT('Ctrl Pts',(-0.59510289473619,-0.400539853271216,
-0.077316548567853));
#10622=CARTESIAN_POINT('Ctrl Pts',(-0.591804743154611,-0.422684184324257,
-0.0994608796208942));
#10623=CARTESIAN_POINT('Ctrl Pts',(-0.590038488226116,-0.436709004341607,
-0.109073016834181));
#10624=CARTESIAN_POINT('Ctrl Pts',(-0.587534197873268,-0.467492086231842,
-0.121843784097853));
#10625=CARTESIAN_POINT('Ctrl Pts',(-0.586834729715275,-0.484254474936005,
-0.125));
#10626=CARTESIAN_POINT('Ctrl Pts',(-0.586834729715275,-0.5,-0.125));
#10627=CARTESIAN_POINT('',(0.586834729715275,-0.5,-0.125));
#10628=CARTESIAN_POINT('',(0.586834729715275,-0.5,0.125));
#10629=CARTESIAN_POINT('Ctrl Pts',(0.586834729715275,-0.5,-0.125));
#10630=CARTESIAN_POINT('Ctrl Pts',(0.586834729715275,-0.484254474936005,
-0.125));
#10631=CARTESIAN_POINT('Ctrl Pts',(0.587534197873268,-0.467492086231842,
-0.121843784097853));
#10632=CARTESIAN_POINT('Ctrl Pts',(0.590038488226116,-0.436709004341607,
-0.109073016834181));
#10633=CARTESIAN_POINT('Ctrl Pts',(0.591804743154611,-0.422684184324257,
-0.0994608796208941));
#10634=CARTESIAN_POINT('Ctrl Pts',(0.59510289473619,-0.400539853271216,
-0.0773165485678529));
#10635=CARTESIAN_POINT('Ctrl Pts',(0.596852269967858,-0.390927142361291,
-0.0632914182239686));
#10636=CARTESIAN_POINT('Ctrl Pts',(0.599317707212167,-0.378155958502111,
-0.0325072544867633));
#10637=CARTESIAN_POINT('Ctrl Pts',(0.6,-0.375,-0.0157444828659572));
#10638=CARTESIAN_POINT('Ctrl Pts',(0.6,-0.375,0.0157444828659573));
#10639=CARTESIAN_POINT('Ctrl Pts',(0.599317707212167,-0.378155958502111,
0.0325072544867635));
#10640=CARTESIAN_POINT('Ctrl Pts',(0.596852269967858,-0.390927142361291,
0.0632914182239687));
#10641=CARTESIAN_POINT('Ctrl Pts',(0.59510289473619,-0.400539853271216,
0.0773165485678531));
#10642=CARTESIAN_POINT('Ctrl Pts',(0.591804743154611,-0.422684184324257,
0.0994608796208942));
#10643=CARTESIAN_POINT('Ctrl Pts',(0.590038488226116,-0.436709004341607,
0.109073016834181));
#10644=CARTESIAN_POINT('Ctrl Pts',(0.587534197873268,-0.467492086231842,
0.121843784097853));
#10645=CARTESIAN_POINT('Ctrl Pts',(0.586834729715275,-0.484254474936005,
0.125));
#10646=CARTESIAN_POINT('Ctrl Pts',(0.586834729715275,-0.5,0.125));
#10647=CARTESIAN_POINT('Ctrl Pts',(0.586834729715275,-0.5,0.125));
#10648=CARTESIAN_POINT('Ctrl Pts',(0.586834729715275,-0.515745525063995,
0.125));
#10649=CARTESIAN_POINT('Ctrl Pts',(0.587534197873268,-0.532507913768158,
0.121843784097853));
#10650=CARTESIAN_POINT('Ctrl Pts',(0.590038488226116,-0.563290995658393,
0.109073016834181));
#10651=CARTESIAN_POINT('Ctrl Pts',(0.591804743154611,-0.577315815675743,
0.0994608796208942));
#10652=CARTESIAN_POINT('Ctrl Pts',(0.59510289473619,-0.599460146728784,
0.077316548567853));
#10653=CARTESIAN_POINT('Ctrl Pts',(0.596852269967858,-0.609072857638709,
0.0632914182239688));
#10654=CARTESIAN_POINT('Ctrl Pts',(0.599317707212167,-0.621844041497889,
0.0325072544867635));
#10655=CARTESIAN_POINT('Ctrl Pts',(0.6,-0.625,0.0157444828659573));
#10656=CARTESIAN_POINT('Ctrl Pts',(0.6,-0.625,-0.0157444828659572));
#10657=CARTESIAN_POINT('Ctrl Pts',(0.599317707212167,-0.621844041497889,
-0.0325072544867633));
#10658=CARTESIAN_POINT('Ctrl Pts',(0.596852269967858,-0.609072857638709,
-0.0632914182239685));
#10659=CARTESIAN_POINT('Ctrl Pts',(0.59510289473619,-0.599460146728784,
-0.077316548567853));
#10660=CARTESIAN_POINT('Ctrl Pts',(0.591804743154611,-0.577315815675743,
-0.0994608796208941));
#10661=CARTESIAN_POINT('Ctrl Pts',(0.590038488226116,-0.563290995658393,
-0.10907301683418));
#10662=CARTESIAN_POINT('Ctrl Pts',(0.587534197873268,-0.532507913768158,
-0.121843784097853));
#10663=CARTESIAN_POINT('Ctrl Pts',(0.586834729715275,-0.515745525063995,
-0.125));
#10664=CARTESIAN_POINT('Ctrl Pts',(0.586834729715275,-0.5,-0.125));
#10665=CARTESIAN_POINT('Origin',(0.,-0.5,0.));
#10666=CARTESIAN_POINT('',(-1.,-0.375,-6.12323399573677E-17));
#10667=CARTESIAN_POINT('',(-0.992156741649222,-0.5,0.125));
#10668=CARTESIAN_POINT('Ctrl Pts',(-1.,-0.375,-1.00613961606655E-16));
#10669=CARTESIAN_POINT('Ctrl Pts',(-1.,-0.375,0.0157128711428661));
#10670=CARTESIAN_POINT('Ctrl Pts',(-0.999591823858855,-0.378143583103513,
0.0324619190698278));
#10671=CARTESIAN_POINT('Ctrl Pts',(-0.998116453123232,-0.390905426591754,
0.0632545375991437));
#10672=CARTESIAN_POINT('Ctrl Pts',(-0.997070068816062,-0.400522781657727,
0.0772994769543643));
#10673=CARTESIAN_POINT('Ctrl Pts',(-0.995102104277285,-0.422700615683787,
0.0994773109804239));
#10674=CARTESIAN_POINT('Ctrl Pts',(-0.994052129228928,-0.436745514765346,
0.109094593469654));
#10675=CARTESIAN_POINT('Ctrl Pts',(-0.99256853061881,-0.467537996927464,
0.121856383722779));
#10676=CARTESIAN_POINT('Ctrl Pts',(-0.992156741649222,-0.484286997589363,
0.125));
#10677=CARTESIAN_POINT('Ctrl Pts',(-0.992156741649222,-0.5,0.125));
#10678=CARTESIAN_POINT('',(-1.,-0.625,-6.12323399573677E-17));
#10679=CARTESIAN_POINT('Ctrl Pts',(-1.,-0.625,-4.5102810375397E-17));
#10680=CARTESIAN_POINT('Ctrl Pts',(-1.,-0.625,-0.0157128711428662));
#10681=CARTESIAN_POINT('Ctrl Pts',(-0.999591823858855,-0.621856416896487,
-0.032461919069828));
#10682=CARTESIAN_POINT('Ctrl Pts',(-0.998116453123232,-0.609094573408246,
-0.0632545375991439));
#10683=CARTESIAN_POINT('Ctrl Pts',(-0.997070068816062,-0.599477218342273,
-0.0772994769543645));
#10684=CARTESIAN_POINT('Ctrl Pts',(-0.995102104277285,-0.577299384316213,
-0.0994773109804241));
#10685=CARTESIAN_POINT('Ctrl Pts',(-0.994052129228928,-0.563254485234654,
-0.109094593469655));
#10686=CARTESIAN_POINT('Ctrl Pts',(-0.99256853061881,-0.532462003072536,
-0.121856383722779));
#10687=CARTESIAN_POINT('Ctrl Pts',(-0.992156741649221,-0.515713002410637,
-0.125));
#10688=CARTESIAN_POINT('Ctrl Pts',(-0.992156741649221,-0.484286997589363,
-0.125));
#10689=CARTESIAN_POINT('Ctrl Pts',(-0.99256853061881,-0.467537996927464,
-0.121856383722779));
#10690=CARTESIAN_POINT('Ctrl Pts',(-0.994052129228928,-0.436745514765346,
-0.109094593469655));
#10691=CARTESIAN_POINT('Ctrl Pts',(-0.995102104277285,-0.422700615683787,
-0.0994773109804241));
#10692=CARTESIAN_POINT('Ctrl Pts',(-0.997070068816062,-0.400522781657728,
-0.0772994769543645));
#10693=CARTESIAN_POINT('Ctrl Pts',(-0.998116453123232,-0.390905426591754,
-0.063254537599144));
#10694=CARTESIAN_POINT('Ctrl Pts',(-0.999591823858855,-0.378143583103513,
-0.0324619190698281));
#10695=CARTESIAN_POINT('Ctrl Pts',(-1.,-0.375,-0.0157128711428663));
#10696=CARTESIAN_POINT('Ctrl Pts',(-1.,-0.375,-9.36750677027476E-17));
#10697=CARTESIAN_POINT('Ctrl Pts',(-0.992156741649222,-0.5,0.125));
#10698=CARTESIAN_POINT('Ctrl Pts',(-0.992156741649222,-0.515713002410637,
0.125));
#10699=CARTESIAN_POINT('Ctrl Pts',(-0.99256853061881,-0.532462003072536,
0.121856383722779));
#10700=CARTESIAN_POINT('Ctrl Pts',(-0.994052129228928,-0.563254485234654,
0.109094593469654));
#10701=CARTESIAN_POINT('Ctrl Pts',(-0.995102104277285,-0.577299384316213,
0.0994773109804241));
#10702=CARTESIAN_POINT('Ctrl Pts',(-0.997070068816062,-0.599477218342273,
0.0772994769543644));
#10703=CARTESIAN_POINT('Ctrl Pts',(-0.998116453123232,-0.609094573408246,
0.0632545375991438));
#10704=CARTESIAN_POINT('Ctrl Pts',(-0.999591823858855,-0.621856416896487,
0.0324619190698279));
#10705=CARTESIAN_POINT('Ctrl Pts',(-1.,-0.625,0.0157128711428661));
#10706=CARTESIAN_POINT('Ctrl Pts',(-1.,-0.625,-4.85722573273506E-17));
#10707=CARTESIAN_POINT('',(-7.65404249467096E-18,-0.5,0.125));
#10708=CARTESIAN_POINT('Origin',(0.,-0.5,0.));
#10709=CARTESIAN_POINT('',(0.992156741649222,-0.5,0.125));
#10710=CARTESIAN_POINT('',(-7.65404249467096E-18,-0.5,0.125));
#10711=CARTESIAN_POINT('',(1.,-0.625,6.12323399573677E-17));
#10712=CARTESIAN_POINT('Ctrl Pts',(1.,-0.625,7.28583859910259E-17));
#10713=CARTESIAN_POINT('Ctrl Pts',(1.,-0.625,0.0157128711428663));
#10714=CARTESIAN_POINT('Ctrl Pts',(0.999591823858855,-0.621856416896487,
0.032461919069828));
#10715=CARTESIAN_POINT('Ctrl Pts',(0.998116453123232,-0.609094573408246,
0.0632545375991439));
#10716=CARTESIAN_POINT('Ctrl Pts',(0.997070068816062,-0.599477218342273,
0.0772994769543645));
#10717=CARTESIAN_POINT('Ctrl Pts',(0.995102104277285,-0.577299384316213,
0.0994773109804242));
#10718=CARTESIAN_POINT('Ctrl Pts',(0.994052129228928,-0.563254485234654,
0.109094593469655));
#10719=CARTESIAN_POINT('Ctrl Pts',(0.99256853061881,-0.532462003072536,
0.121856383722779));
#10720=CARTESIAN_POINT('Ctrl Pts',(0.992156741649222,-0.515713002410637,
0.125));
#10721=CARTESIAN_POINT('Ctrl Pts',(0.992156741649222,-0.5,0.125));
#10722=CARTESIAN_POINT('',(1.,-0.375,6.12323399573677E-17));
#10723=CARTESIAN_POINT('Ctrl Pts',(1.,-0.375,2.08166817117217E-17));
#10724=CARTESIAN_POINT('Ctrl Pts',(1.,-0.375,-0.0157128711428662));
#10725=CARTESIAN_POINT('Ctrl Pts',(0.999591823858855,-0.378143583103513,
-0.032461919069828));
#10726=CARTESIAN_POINT('Ctrl Pts',(0.998116453123232,-0.390905426591754,
-0.0632545375991438));
#10727=CARTESIAN_POINT('Ctrl Pts',(0.997070068816062,-0.400522781657728,
-0.0772994769543644));
#10728=CARTESIAN_POINT('Ctrl Pts',(0.995102104277285,-0.422700615683787,
-0.099477310980424));
#10729=CARTESIAN_POINT('Ctrl Pts',(0.994052129228928,-0.436745514765346,
-0.109094593469654));
#10730=CARTESIAN_POINT('Ctrl Pts',(0.99256853061881,-0.467537996927464,
-0.121856383722779));
#10731=CARTESIAN_POINT('Ctrl Pts',(0.992156741649222,-0.484286997589363,
-0.125));
#10732=CARTESIAN_POINT('Ctrl Pts',(0.992156741649222,-0.515713002410637,
-0.125));
#10733=CARTESIAN_POINT('Ctrl Pts',(0.99256853061881,-0.532462003072536,
-0.121856383722779));
#10734=CARTESIAN_POINT('Ctrl Pts',(0.994052129228928,-0.563254485234654,
-0.109094593469654));
#10735=CARTESIAN_POINT('Ctrl Pts',(0.995102104277285,-0.577299384316213,
-0.099477310980424));
#10736=CARTESIAN_POINT('Ctrl Pts',(0.997070068816062,-0.599477218342273,
-0.0772994769543643));
#10737=CARTESIAN_POINT('Ctrl Pts',(0.998116453123232,-0.609094573408246,
-0.0632545375991438));
#10738=CARTESIAN_POINT('Ctrl Pts',(0.999591823858855,-0.621856416896487,
-0.0324619190698279));
#10739=CARTESIAN_POINT('Ctrl Pts',(1.,-0.625,-0.0157128711428661));
#10740=CARTESIAN_POINT('Ctrl Pts',(1.,-0.625,8.32667268468867E-17));
#10741=CARTESIAN_POINT('Ctrl Pts',(0.992156741649222,-0.5,0.125));
#10742=CARTESIAN_POINT('Ctrl Pts',(0.992156741649222,-0.484286997589363,
0.125));
#10743=CARTESIAN_POINT('Ctrl Pts',(0.99256853061881,-0.467537996927464,
0.121856383722779));
#10744=CARTESIAN_POINT('Ctrl Pts',(0.994052129228928,-0.436745514765346,
0.109094593469654));
#10745=CARTESIAN_POINT('Ctrl Pts',(0.995102104277285,-0.422700615683787,
0.0994773109804241));
#10746=CARTESIAN_POINT('Ctrl Pts',(0.997070068816062,-0.400522781657727,
0.0772994769543644));
#10747=CARTESIAN_POINT('Ctrl Pts',(0.998116453123232,-0.390905426591754,
0.0632545375991438));
#10748=CARTESIAN_POINT('Ctrl Pts',(0.999591823858855,-0.378143583103513,
0.0324619190698279));
#10749=CARTESIAN_POINT('Ctrl Pts',(1.,-0.375,0.0157128711428662));
#10750=CARTESIAN_POINT('Ctrl Pts',(1.,-0.375,2.77555756156289E-17));
#10751=CARTESIAN_POINT('Origin',(0.,-0.1,0.));
#10752=CARTESIAN_POINT('',(-1.,-0.9,1.22464679914735E-16));
#10753=CARTESIAN_POINT('Origin',(0.,-0.9,0.));
#10754=CARTESIAN_POINT('',(-1.,-0.1,-1.22464679914735E-16));
#10755=CARTESIAN_POINT('',(-1.,-0.1,1.22464679914735E-16));
#10756=CARTESIAN_POINT('',(-1.,-0.1,-1.22464679914735E-16));
#10757=CARTESIAN_POINT('Origin',(0.,-0.1,0.));
#10758=CARTESIAN_POINT('',(0.,-0.625,-1.));
#10759=CARTESIAN_POINT('',(0.,-0.375,-1.));
#10760=CARTESIAN_POINT('Ctrl Pts',(-2.08166817117217E-17,-0.625,-1.));
#10761=CARTESIAN_POINT('Ctrl Pts',(0.0157128711428662,-0.625,-1.));
#10762=CARTESIAN_POINT('Ctrl Pts',(0.0324619190698279,-0.621856416896487,
-0.999591823858855));
#10763=CARTESIAN_POINT('Ctrl Pts',(0.0632545375991438,-0.609094573408246,
-0.998116453123232));
#10764=CARTESIAN_POINT('Ctrl Pts',(0.0772994769543644,-0.599477218342273,
-0.997070068816062));
#10765=CARTESIAN_POINT('Ctrl Pts',(0.0994773109804241,-0.577299384316213,
-0.995102104277285));
#10766=CARTESIAN_POINT('Ctrl Pts',(0.109094593469654,-0.563254485234654,
-0.994052129228928));
#10767=CARTESIAN_POINT('Ctrl Pts',(0.121856383722779,-0.532462003072536,
-0.99256853061881));
#10768=CARTESIAN_POINT('Ctrl Pts',(0.125,-0.515713002410637,-0.992156741649221));
#10769=CARTESIAN_POINT('Ctrl Pts',(0.125,-0.484286997589363,-0.992156741649221));
#10770=CARTESIAN_POINT('Ctrl Pts',(0.121856383722779,-0.467537996927464,
-0.99256853061881));
#10771=CARTESIAN_POINT('Ctrl Pts',(0.109094593469654,-0.436745514765346,
-0.994052129228928));
#10772=CARTESIAN_POINT('Ctrl Pts',(0.0994773109804241,-0.422700615683787,
-0.995102104277285));
#10773=CARTESIAN_POINT('Ctrl Pts',(0.0772994769543645,-0.400522781657728,
-0.997070068816062));
#10774=CARTESIAN_POINT('Ctrl Pts',(0.0632545375991439,-0.390905426591754,
-0.998116453123232));
#10775=CARTESIAN_POINT('Ctrl Pts',(0.032461919069828,-0.378143583103513,
-0.999591823858855));
#10776=CARTESIAN_POINT('Ctrl Pts',(0.0157128711428662,-0.375,-1.));
#10777=CARTESIAN_POINT('Ctrl Pts',(3.81639164714898E-17,-0.375,-1.));
#10778=CARTESIAN_POINT('',(-0.125,-0.5,-0.992156741649222));
#10779=CARTESIAN_POINT('Ctrl Pts',(4.5102810375397E-17,-0.375,-1.));
#10780=CARTESIAN_POINT('Ctrl Pts',(-0.0157128711428661,-0.375,-1.));
#10781=CARTESIAN_POINT('Ctrl Pts',(-0.0324619190698279,-0.378143583103513,
-0.999591823858855));
#10782=CARTESIAN_POINT('Ctrl Pts',(-0.0632545375991437,-0.390905426591754,
-0.998116453123232));
#10783=CARTESIAN_POINT('Ctrl Pts',(-0.0772994769543643,-0.400522781657727,
-0.997070068816062));
#10784=CARTESIAN_POINT('Ctrl Pts',(-0.099477310980424,-0.422700615683787,
-0.995102104277285));
#10785=CARTESIAN_POINT('Ctrl Pts',(-0.109094593469654,-0.436745514765346,
-0.994052129228928));
#10786=CARTESIAN_POINT('Ctrl Pts',(-0.121856383722779,-0.467537996927464,
-0.99256853061881));
#10787=CARTESIAN_POINT('Ctrl Pts',(-0.125,-0.484286997589363,-0.992156741649222));
#10788=CARTESIAN_POINT('Ctrl Pts',(-0.125,-0.5,-0.992156741649222));
#10789=CARTESIAN_POINT('Ctrl Pts',(-0.125,-0.5,-0.992156741649222));
#10790=CARTESIAN_POINT('Ctrl Pts',(-0.125,-0.515713002410637,-0.992156741649222));
#10791=CARTESIAN_POINT('Ctrl Pts',(-0.121856383722779,-0.532462003072536,
-0.99256853061881));
#10792=CARTESIAN_POINT('Ctrl Pts',(-0.109094593469654,-0.563254485234654,
-0.994052129228928));
#10793=CARTESIAN_POINT('Ctrl Pts',(-0.0994773109804241,-0.577299384316213,
-0.995102104277285));
#10794=CARTESIAN_POINT('Ctrl Pts',(-0.0772994769543644,-0.599477218342273,
-0.997070068816062));
#10795=CARTESIAN_POINT('Ctrl Pts',(-0.0632545375991439,-0.609094573408246,
-0.998116453123232));
#10796=CARTESIAN_POINT('Ctrl Pts',(-0.032461919069828,-0.621856416896487,
-0.999591823858855));
#10797=CARTESIAN_POINT('Ctrl Pts',(-0.0157128711428662,-0.625,-1.));
#10798=CARTESIAN_POINT('Ctrl Pts',(-1.38777878078145E-17,-0.625,-1.));
#10799=CARTESIAN_POINT('',(0.,-0.375,1.));
#10800=CARTESIAN_POINT('',(0.,-0.625,1.));
#10801=CARTESIAN_POINT('Ctrl Pts',(4.16333634234434E-17,-0.375,1.));
#10802=CARTESIAN_POINT('Ctrl Pts',(0.0157128711428662,-0.375,1.));
#10803=CARTESIAN_POINT('Ctrl Pts',(0.032461919069828,-0.378143583103513,
0.999591823858855));
#10804=CARTESIAN_POINT('Ctrl Pts',(0.0632545375991439,-0.390905426591754,
0.998116453123232));
#10805=CARTESIAN_POINT('Ctrl Pts',(0.0772994769543644,-0.400522781657728,
0.997070068816062));
#10806=CARTESIAN_POINT('Ctrl Pts',(0.0994773109804241,-0.422700615683787,
0.995102104277285));
#10807=CARTESIAN_POINT('Ctrl Pts',(0.109094593469654,-0.436745514765346,
0.994052129228928));
#10808=CARTESIAN_POINT('Ctrl Pts',(0.121856383722779,-0.467537996927464,
0.99256853061881));
#10809=CARTESIAN_POINT('Ctrl Pts',(0.125,-0.484286997589363,0.992156741649222));
#10810=CARTESIAN_POINT('Ctrl Pts',(0.125,-0.515713002410637,0.992156741649222));
#10811=CARTESIAN_POINT('Ctrl Pts',(0.121856383722779,-0.532462003072536,
0.99256853061881));
#10812=CARTESIAN_POINT('Ctrl Pts',(0.109094593469655,-0.563254485234654,
0.994052129228928));
#10813=CARTESIAN_POINT('Ctrl Pts',(0.0994773109804241,-0.577299384316213,
0.995102104277285));
#10814=CARTESIAN_POINT('Ctrl Pts',(0.0772994769543644,-0.599477218342273,
0.997070068816062));
#10815=CARTESIAN_POINT('Ctrl Pts',(0.0632545375991438,-0.609094573408246,
0.998116453123232));
#10816=CARTESIAN_POINT('Ctrl Pts',(0.0324619190698279,-0.621856416896487,
0.999591823858855));
#10817=CARTESIAN_POINT('Ctrl Pts',(0.0157128711428662,-0.625,1.));
#10818=CARTESIAN_POINT('Ctrl Pts',(-1.73472347597681E-17,-0.625,1.));
#10819=CARTESIAN_POINT('',(-0.125,-0.5,0.992156741649222));
#10820=CARTESIAN_POINT('Ctrl Pts',(-1.73472347597681E-17,-0.625,1.));
#10821=CARTESIAN_POINT('Ctrl Pts',(-0.0157128711428662,-0.625,1.));
#10822=CARTESIAN_POINT('Ctrl Pts',(-0.032461919069828,-0.621856416896487,
0.999591823858855));
#10823=CARTESIAN_POINT('Ctrl Pts',(-0.0632545375991439,-0.609094573408246,
0.998116453123232));
#10824=CARTESIAN_POINT('Ctrl Pts',(-0.0772994769543645,-0.599477218342273,
0.997070068816062));
#10825=CARTESIAN_POINT('Ctrl Pts',(-0.0994773109804241,-0.577299384316213,
0.995102104277285));
#10826=CARTESIAN_POINT('Ctrl Pts',(-0.109094593469654,-0.563254485234654,
0.994052129228928));
#10827=CARTESIAN_POINT('Ctrl Pts',(-0.121856383722779,-0.532462003072536,
0.99256853061881));
#10828=CARTESIAN_POINT('Ctrl Pts',(-0.125,-0.515713002410637,0.992156741649222));
#10829=CARTESIAN_POINT('Ctrl Pts',(-0.125,-0.5,0.992156741649222));
#10830=CARTESIAN_POINT('Ctrl Pts',(-0.125,-0.5,0.992156741649222));
#10831=CARTESIAN_POINT('Ctrl Pts',(-0.125,-0.484286997589363,0.992156741649222));
#10832=CARTESIAN_POINT('Ctrl Pts',(-0.121856383722779,-0.467537996927464,
0.99256853061881));
#10833=CARTESIAN_POINT('Ctrl Pts',(-0.109094593469654,-0.436745514765346,
0.994052129228928));
#10834=CARTESIAN_POINT('Ctrl Pts',(-0.099477310980424,-0.422700615683787,
0.995102104277285));
#10835=CARTESIAN_POINT('Ctrl Pts',(-0.0772994769543643,-0.400522781657727,
0.997070068816062));
#10836=CARTESIAN_POINT('Ctrl Pts',(-0.0632545375991438,-0.390905426591754,
0.998116453123232));
#10837=CARTESIAN_POINT('Ctrl Pts',(-0.0324619190698279,-0.378143583103513,
0.999591823858855));
#10838=CARTESIAN_POINT('Ctrl Pts',(-0.0157128711428661,-0.375,1.));
#10839=CARTESIAN_POINT('Ctrl Pts',(4.5102810375397E-17,-0.375,1.));
#10840=CARTESIAN_POINT('Origin',(0.,-0.5,0.));
#10841=CARTESIAN_POINT('',(-0.125,-0.5,0.));
#10842=CARTESIAN_POINT('Origin',(0.,-0.5,0.));
#10843=CARTESIAN_POINT('',(-0.125,-0.5,0.));
#10844=CARTESIAN_POINT('Origin',(0.,-0.9,0.));
#10845=CARTESIAN_POINT('Origin',(0.,0.,0.));
#10846=CARTESIAN_POINT('',(-1.4,0.,1.71450551880629E-16));
#10847=CARTESIAN_POINT('Origin',(0.,0.,0.));
#10848=CARTESIAN_POINT('',(1.23958209161204,0.,0.143317017690053));
#10849=CARTESIAN_POINT('',(1.22320001975977,0.,0.246749348660852));
#10850=CARTESIAN_POINT('Origin',(1.21321664662686,0.,0.192154639568406));
#10851=CARTESIAN_POINT('',(1.20190105810224,0.,0.335465908756113));
#10852=CARTESIAN_POINT('Origin',(0.,0.,0.));
#10853=CARTESIAN_POINT('',(1.16954029537568,0.,0.435062095450087));
#10854=CARTESIAN_POINT('Origin',(1.1682203282434,0.,0.379577794185952));
#10855=CARTESIAN_POINT('',(1.13462523166105,0.,0.519354515801077));
#10856=CARTESIAN_POINT('Origin',(0.,0.,0.));
#10857=CARTESIAN_POINT('',(1.08708260743774,0.,0.612662169561029));
#10858=CARTESIAN_POINT('Origin',(1.0944585482776,0.,0.557654483764164));
#10859=CARTESIAN_POINT('',(1.0394111664111,0.,0.690454891028201));
#10860=CARTESIAN_POINT('Origin',(0.,0.,0.));
#10861=CARTESIAN_POINT('',(0.977857337884349,0.,0.775176467748211));
#10862=CARTESIAN_POINT('Origin',(0.993747566553533,0.,0.72199986920298));
#10863=CARTESIAN_POINT('',(0.918603348636233,0.,0.844553975349804));
#10864=CARTESIAN_POINT('Origin',(0.,0.,0.));
#10865=CARTESIAN_POINT('',(0.844553975349804,0.,0.918603348636233));
#10866=CARTESIAN_POINT('Origin',(0.86856722168183,0.,0.86856722168183));
#10867=CARTESIAN_POINT('',(0.775176467748211,0.,0.977857337884349));
#10868=CARTESIAN_POINT('Origin',(0.,0.,0.));
#10869=CARTESIAN_POINT('',(0.690454891028201,0.,1.0394111664111));
#10870=CARTESIAN_POINT('Origin',(0.721999869202979,0.,0.993747566553533));
#10871=CARTESIAN_POINT('',(0.612662169561028,0.,1.08708260743774));
#10872=CARTESIAN_POINT('Origin',(0.,0.,0.));
#10873=CARTESIAN_POINT('',(0.519354515801077,0.,1.13462523166105));
#10874=CARTESIAN_POINT('Origin',(0.557654483764164,0.,1.0944585482776));
#10875=CARTESIAN_POINT('',(0.435062095450087,0.,1.16954029537568));
#10876=CARTESIAN_POINT('Origin',(0.,0.,0.));
#10877=CARTESIAN_POINT('',(0.335465908756113,0.,1.20190105810224));
#10878=CARTESIAN_POINT('Origin',(0.379577794185951,0.,1.1682203282434));
#10879=CARTESIAN_POINT('',(0.246749348660851,0.,1.22320001975977));
#10880=CARTESIAN_POINT('Origin',(0.,0.,0.));
#10881=CARTESIAN_POINT('',(0.143317017690053,0.,1.23958209161204));
#10882=CARTESIAN_POINT('Origin',(0.192154639568406,0.,1.21321664662686));
#10883=CARTESIAN_POINT('',(0.0523608139934478,0.,1.24674050008925));
#10884=CARTESIAN_POINT('Origin',(0.,0.,0.));
#10885=CARTESIAN_POINT('',(-0.0523608139934483,0.,1.24674050008925));
#10886=CARTESIAN_POINT('Origin',(-2.25642313758905E-16,0.,1.22833954473516));
#10887=CARTESIAN_POINT('',(-0.143317017690053,0.,1.23958209161204));
#10888=CARTESIAN_POINT('Origin',(0.,0.,0.));
#10889=CARTESIAN_POINT('',(-0.246749348660852,0.,1.22320001975977));
#10890=CARTESIAN_POINT('Origin',(-0.192154639568406,0.,1.21321664662686));
#10891=CARTESIAN_POINT('',(-0.335465908756113,0.,1.20190105810224));
#10892=CARTESIAN_POINT('Origin',(0.,0.,0.));
#10893=CARTESIAN_POINT('',(-0.435062095450087,0.,1.16954029537568));
#10894=CARTESIAN_POINT('Origin',(-0.379577794185951,0.,1.1682203282434));
#10895=CARTESIAN_POINT('',(-0.519354515801077,0.,1.13462523166105));
#10896=CARTESIAN_POINT('Origin',(0.,0.,0.));
#10897=CARTESIAN_POINT('',(-0.612662169561029,0.,1.08708260743774));
#10898=CARTESIAN_POINT('Origin',(-0.557654483764164,0.,1.0944585482776));
#10899=CARTESIAN_POINT('',(-0.690454891028201,0.,1.0394111664111));
#10900=CARTESIAN_POINT('Origin',(0.,0.,0.));
#10901=CARTESIAN_POINT('',(-0.775176467748211,0.,0.977857337884349));
#10902=CARTESIAN_POINT('Origin',(-0.721999869202979,0.,0.993747566553533));
#10903=CARTESIAN_POINT('',(-0.844553975349804,0.,0.918603348636233));
#10904=CARTESIAN_POINT('Origin',(0.,0.,0.));
#10905=CARTESIAN_POINT('',(-0.918603348636233,0.,0.844553975349804));
#10906=CARTESIAN_POINT('Origin',(-0.86856722168183,0.,0.86856722168183));
#10907=CARTESIAN_POINT('',(-0.977857337884348,0.,0.775176467748211));
#10908=CARTESIAN_POINT('Origin',(0.,0.,0.));
#10909=CARTESIAN_POINT('',(-1.0394111664111,0.,0.690454891028201));
#10910=CARTESIAN_POINT('Origin',(-0.993747566553533,0.,0.721999869202979));
#10911=CARTESIAN_POINT('',(-1.08708260743774,0.,0.612662169561028));
#10912=CARTESIAN_POINT('Origin',(0.,0.,0.));
#10913=CARTESIAN_POINT('',(-1.13462523166105,0.,0.519354515801077));
#10914=CARTESIAN_POINT('Origin',(-1.0944585482776,0.,0.557654483764164));
#10915=CARTESIAN_POINT('',(-1.16954029537568,0.,0.435062095450087));
#10916=CARTESIAN_POINT('Origin',(0.,0.,0.));
#10917=CARTESIAN_POINT('',(-1.20190105810224,0.,0.335465908756113));
#10918=CARTESIAN_POINT('Origin',(-1.1682203282434,0.,0.379577794185951));
#10919=CARTESIAN_POINT('',(-1.22320001975977,0.,0.246749348660851));
#10920=CARTESIAN_POINT('Origin',(0.,0.,0.));
#10921=CARTESIAN_POINT('',(-1.23958209161204,0.,0.143317017690053));
#10922=CARTESIAN_POINT('Origin',(-1.21321664662686,0.,0.192154639568406));
#10923=CARTESIAN_POINT('',(-1.24674050008925,0.,0.0523608139934479));
#10924=CARTESIAN_POINT('Origin',(0.,0.,0.));
#10925=CARTESIAN_POINT('',(-1.24674050008925,0.,-0.0523608139934482));
#10926=CARTESIAN_POINT('Origin',(-1.22833954473516,0.,-1.50428209172603E-16));
#10927=CARTESIAN_POINT('',(-1.23958209161204,0.,-0.143317017690053));
#10928=CARTESIAN_POINT('Origin',(0.,0.,0.));
#10929=CARTESIAN_POINT('',(-1.22320001975977,0.,-0.246749348660852));
#10930=CARTESIAN_POINT('Origin',(-1.21321664662686,0.,-0.192154639568406));
#10931=CARTESIAN_POINT('',(-1.20190105810224,0.,-0.335465908756113));
#10932=CARTESIAN_POINT('Origin',(0.,0.,0.));
#10933=CARTESIAN_POINT('',(-1.16954029537568,0.,-0.435062095450087));
#10934=CARTESIAN_POINT('Origin',(-1.1682203282434,0.,-0.379577794185951));
#10935=CARTESIAN_POINT('',(-1.13462523166105,0.,-0.519354515801077));
#10936=CARTESIAN_POINT('Origin',(0.,0.,0.));
#10937=CARTESIAN_POINT('',(-1.08708260743774,0.,-0.612662169561029));
#10938=CARTESIAN_POINT('Origin',(-1.0944585482776,0.,-0.557654483764164));
#10939=CARTESIAN_POINT('',(-1.0394111664111,0.,-0.690454891028201));
#10940=CARTESIAN_POINT('Origin',(0.,0.,0.));
#10941=CARTESIAN_POINT('',(-0.977857337884349,0.,-0.775176467748211));
#10942=CARTESIAN_POINT('Origin',(-0.993747566553533,0.,-0.721999869202979));
#10943=CARTESIAN_POINT('',(-0.918603348636233,0.,-0.844553975349804));
#10944=CARTESIAN_POINT('Origin',(0.,0.,0.));
#10945=CARTESIAN_POINT('',(-0.844553975349804,0.,-0.918603348636233));
#10946=CARTESIAN_POINT('Origin',(-0.86856722168183,0.,-0.86856722168183));
#10947=CARTESIAN_POINT('',(-0.775176467748211,0.,-0.977857337884348));
#10948=CARTESIAN_POINT('Origin',(0.,0.,0.));
#10949=CARTESIAN_POINT('',(-0.690454891028201,0.,-1.0394111664111));
#10950=CARTESIAN_POINT('Origin',(-0.721999869202979,0.,-0.993747566553533));
#10951=CARTESIAN_POINT('',(-0.612662169561028,0.,-1.08708260743774));
#10952=CARTESIAN_POINT('Origin',(0.,0.,0.));
#10953=CARTESIAN_POINT('',(-0.519354515801077,0.,-1.13462523166105));
#10954=CARTESIAN_POINT('Origin',(-0.557654483764164,0.,-1.0944585482776));
#10955=CARTESIAN_POINT('',(-0.435062095450087,0.,-1.16954029537568));
#10956=CARTESIAN_POINT('Origin',(0.,0.,0.));
#10957=CARTESIAN_POINT('',(-0.335465908756113,0.,-1.20190105810224));
#10958=CARTESIAN_POINT('Origin',(-0.379577794185951,0.,-1.1682203282434));
#10959=CARTESIAN_POINT('',(-0.246749348660852,0.,-1.22320001975977));
#10960=CARTESIAN_POINT('Origin',(0.,0.,0.));
#10961=CARTESIAN_POINT('',(-0.143317017690053,0.,-1.23958209161204));
#10962=CARTESIAN_POINT('Origin',(-0.192154639568406,0.,-1.21321664662686));
#10963=CARTESIAN_POINT('',(-0.0523608139934479,0.,-1.24674050008925));
#10964=CARTESIAN_POINT('Origin',(0.,0.,0.));
#10965=CARTESIAN_POINT('',(0.0523608139934481,0.,-1.24674050008925));
#10966=CARTESIAN_POINT('Origin',(7.52141045863017E-17,0.,-1.22833954473516));
#10967=CARTESIAN_POINT('',(0.143317017690053,0.,-1.23958209161204));
#10968=CARTESIAN_POINT('Origin',(0.,0.,0.));
#10969=CARTESIAN_POINT('',(0.246749348660852,0.,-1.22320001975977));
#10970=CARTESIAN_POINT('Origin',(0.192154639568406,0.,-1.21321664662686));
#10971=CARTESIAN_POINT('',(0.335465908756113,0.,-1.20190105810224));
#10972=CARTESIAN_POINT('Origin',(0.,0.,0.));
#10973=CARTESIAN_POINT('',(0.435062095450087,0.,-1.16954029537568));
#10974=CARTESIAN_POINT('Origin',(0.379577794185951,0.,-1.1682203282434));
#10975=CARTESIAN_POINT('',(0.519354515801077,0.,-1.13462523166105));
#10976=CARTESIAN_POINT('Origin',(0.,0.,0.));
#10977=CARTESIAN_POINT('',(0.612662169561028,0.,-1.08708260743774));
#10978=CARTESIAN_POINT('Origin',(0.557654483764164,0.,-1.0944585482776));
#10979=CARTESIAN_POINT('',(0.690454891028201,0.,-1.0394111664111));
#10980=CARTESIAN_POINT('Origin',(0.,0.,0.));
#10981=CARTESIAN_POINT('',(0.775176467748211,0.,-0.977857337884349));
#10982=CARTESIAN_POINT('Origin',(0.721999869202979,0.,-0.993747566553533));
#10983=CARTESIAN_POINT('',(0.844553975349804,0.,-0.918603348636233));
#10984=CARTESIAN_POINT('Origin',(0.,0.,0.));
#10985=CARTESIAN_POINT('',(0.918603348636233,0.,-0.844553975349804));
#10986=CARTESIAN_POINT('Origin',(0.86856722168183,0.,-0.86856722168183));
#10987=CARTESIAN_POINT('',(0.977857337884349,0.,-0.775176467748211));
#10988=CARTESIAN_POINT('Origin',(0.,0.,0.));
#10989=CARTESIAN_POINT('',(1.0394111664111,0.,-0.690454891028201));
#10990=CARTESIAN_POINT('Origin',(0.993747566553533,0.,-0.721999869202979));
#10991=CARTESIAN_POINT('',(1.08708260743774,0.,-0.612662169561028));
#10992=CARTESIAN_POINT('Origin',(0.,0.,0.));
#10993=CARTESIAN_POINT('',(1.13462523166105,0.,-0.519354515801077));
#10994=CARTESIAN_POINT('Origin',(1.0944585482776,0.,-0.557654483764164));
#10995=CARTESIAN_POINT('',(1.16954029537568,0.,-0.43506209545009));
#10996=CARTESIAN_POINT('Origin',(0.,0.,0.));
#10997=CARTESIAN_POINT('',(1.20190105810224,0.,-0.33546590875611));
#10998=CARTESIAN_POINT('Origin',(1.1682203282434,0.,-0.379577794185951));
#10999=CARTESIAN_POINT('',(1.22320001975977,0.,-0.246749348660852));
#11000=CARTESIAN_POINT('Origin',(0.,0.,0.));
#11001=CARTESIAN_POINT('',(1.23958209161204,0.,-0.143317017690053));
#11002=CARTESIAN_POINT('Origin',(1.21321664662686,0.,-0.192154639568406));
#11003=CARTESIAN_POINT('',(1.24674050008925,0.,-0.052360813993451));
#11004=CARTESIAN_POINT('Origin',(0.,0.,0.));
#11005=CARTESIAN_POINT('',(1.24674050008925,0.,0.052360813993451));
#11006=CARTESIAN_POINT('Origin',(1.22833954473516,0.,0.));
#11007=CARTESIAN_POINT('Origin',(0.,0.,0.));
#11008=CARTESIAN_POINT('Origin',(0.,0.,0.));
#11009=CARTESIAN_POINT('',(-1.4,-0.1,1.71450551880629E-16));
#11010=CARTESIAN_POINT('Origin',(0.,-0.1,0.));
#11011=CARTESIAN_POINT('',(-1.4,0.,-1.71450551880629E-16));
#11012=CARTESIAN_POINT('Origin',(0.,-0.1,0.));
#11013=CARTESIAN_POINT('Origin',(0.,0.75,0.));
#11014=CARTESIAN_POINT('',(-1.4,0.75,1.71450551880629E-16));
#11015=CARTESIAN_POINT('Origin',(0.,0.75,0.));
#11016=CARTESIAN_POINT('',(1.22320001975977,0.75,0.246749348660852));
#11017=CARTESIAN_POINT('',(1.23958209161204,0.75,0.143317017690053));
#11018=CARTESIAN_POINT('Origin',(1.21321664662686,0.75,0.192154639568406));
#11019=CARTESIAN_POINT('',(1.24674050008925,0.75,0.052360813993448));
#11020=CARTESIAN_POINT('Origin',(0.,0.75,0.));
#11021=CARTESIAN_POINT('',(1.24674050008925,0.75,-0.052360813993448));
#11022=CARTESIAN_POINT('Origin',(1.22833954473516,0.75,0.));
#11023=CARTESIAN_POINT('',(1.23958209161204,0.75,-0.143317017690053));
#11024=CARTESIAN_POINT('Origin',(0.,0.75,0.));
#11025=CARTESIAN_POINT('',(1.22320001975977,0.75,-0.246749348660852));
#11026=CARTESIAN_POINT('Origin',(1.21321664662686,0.75,-0.192154639568406));
#11027=CARTESIAN_POINT('',(1.20190105810224,0.75,-0.335465908756113));
#11028=CARTESIAN_POINT('Origin',(0.,0.75,0.));
#11029=CARTESIAN_POINT('',(1.16954029537568,0.75,-0.435062095450087));
#11030=CARTESIAN_POINT('Origin',(1.1682203282434,0.75,-0.379577794185951));
#11031=CARTESIAN_POINT('',(1.13462523166105,0.75,-0.519354515801077));
#11032=CARTESIAN_POINT('Origin',(0.,0.75,0.));
#11033=CARTESIAN_POINT('',(1.08708260743774,0.75,-0.612662169561028));
#11034=CARTESIAN_POINT('Origin',(1.0944585482776,0.75,-0.557654483764164));
#11035=CARTESIAN_POINT('',(1.0394111664111,0.75,-0.690454891028201));
#11036=CARTESIAN_POINT('Origin',(0.,0.75,0.));
#11037=CARTESIAN_POINT('',(0.977857337884349,0.75,-0.775176467748211));
#11038=CARTESIAN_POINT('Origin',(0.993747566553533,0.75,-0.721999869202979));
#11039=CARTESIAN_POINT('',(0.918603348636233,0.75,-0.844553975349804));
#11040=CARTESIAN_POINT('Origin',(0.,0.75,0.));
#11041=CARTESIAN_POINT('',(0.844553975349804,0.75,-0.918603348636233));
#11042=CARTESIAN_POINT('Origin',(0.86856722168183,0.75,-0.86856722168183));
#11043=CARTESIAN_POINT('',(0.775176467748211,0.75,-0.977857337884349));
#11044=CARTESIAN_POINT('Origin',(0.,0.75,0.));
#11045=CARTESIAN_POINT('',(0.690454891028201,0.75,-1.0394111664111));
#11046=CARTESIAN_POINT('Origin',(0.721999869202979,0.75,-0.993747566553533));
#11047=CARTESIAN_POINT('',(0.612662169561028,0.75,-1.08708260743774));
#11048=CARTESIAN_POINT('Origin',(0.,0.75,0.));
#11049=CARTESIAN_POINT('',(0.519354515801077,0.75,-1.13462523166105));
#11050=CARTESIAN_POINT('Origin',(0.557654483764164,0.75,-1.0944585482776));
#11051=CARTESIAN_POINT('',(0.435062095450087,0.75,-1.16954029537568));
#11052=CARTESIAN_POINT('Origin',(0.,0.75,0.));
#11053=CARTESIAN_POINT('',(0.335465908756113,0.75,-1.20190105810224));
#11054=CARTESIAN_POINT('Origin',(0.379577794185951,0.75,-1.1682203282434));
#11055=CARTESIAN_POINT('',(0.246749348660852,0.75,-1.22320001975977));
#11056=CARTESIAN_POINT('Origin',(0.,0.75,0.));
#11057=CARTESIAN_POINT('',(0.143317017690053,0.75,-1.23958209161204));
#11058=CARTESIAN_POINT('Origin',(0.192154639568406,0.75,-1.21321664662686));
#11059=CARTESIAN_POINT('',(0.0523608139934481,0.75,-1.24674050008925));
#11060=CARTESIAN_POINT('Origin',(0.,0.75,0.));
#11061=CARTESIAN_POINT('',(-0.0523608139934479,0.75,-1.24674050008925));
#11062=CARTESIAN_POINT('Origin',(7.52141045863017E-17,0.75,-1.22833954473516));
#11063=CARTESIAN_POINT('',(-0.143317017690053,0.75,-1.23958209161204));
#11064=CARTESIAN_POINT('Origin',(0.,0.75,0.));
#11065=CARTESIAN_POINT('',(-0.246749348660852,0.75,-1.22320001975977));
#11066=CARTESIAN_POINT('Origin',(-0.192154639568406,0.75,-1.21321664662686));
#11067=CARTESIAN_POINT('',(-0.335465908756113,0.75,-1.20190105810224));
#11068=CARTESIAN_POINT('Origin',(0.,0.75,0.));
#11069=CARTESIAN_POINT('',(-0.435062095450087,0.75,-1.16954029537568));
#11070=CARTESIAN_POINT('Origin',(-0.379577794185951,0.75,-1.1682203282434));
#11071=CARTESIAN_POINT('',(-0.519354515801077,0.75,-1.13462523166105));
#11072=CARTESIAN_POINT('Origin',(0.,0.75,0.));
#11073=CARTESIAN_POINT('',(-0.612662169561028,0.75,-1.08708260743774));
#11074=CARTESIAN_POINT('Origin',(-0.557654483764164,0.75,-1.0944585482776));
#11075=CARTESIAN_POINT('',(-0.690454891028201,0.75,-1.0394111664111));
#11076=CARTESIAN_POINT('Origin',(0.,0.75,0.));
#11077=CARTESIAN_POINT('',(-0.775176467748211,0.75,-0.977857337884348));
#11078=CARTESIAN_POINT('Origin',(-0.721999869202979,0.75,-0.993747566553533));
#11079=CARTESIAN_POINT('',(-0.844553975349804,0.75,-0.918603348636233));
#11080=CARTESIAN_POINT('Origin',(0.,0.75,0.));
#11081=CARTESIAN_POINT('',(-0.918603348636233,0.75,-0.844553975349804));
#11082=CARTESIAN_POINT('Origin',(-0.86856722168183,0.75,-0.86856722168183));
#11083=CARTESIAN_POINT('',(-0.977857337884349,0.75,-0.775176467748211));
#11084=CARTESIAN_POINT('Origin',(0.,0.75,0.));
#11085=CARTESIAN_POINT('',(-1.0394111664111,0.75,-0.690454891028201));
#11086=CARTESIAN_POINT('Origin',(-0.993747566553533,0.75,-0.721999869202979));
#11087=CARTESIAN_POINT('',(-1.08708260743774,0.75,-0.612662169561029));
#11088=CARTESIAN_POINT('Origin',(0.,0.75,0.));
#11089=CARTESIAN_POINT('',(-1.13462523166105,0.75,-0.519354515801077));
#11090=CARTESIAN_POINT('Origin',(-1.0944585482776,0.75,-0.557654483764164));
#11091=CARTESIAN_POINT('',(-1.16954029537568,0.75,-0.435062095450087));
#11092=CARTESIAN_POINT('Origin',(0.,0.75,0.));
#11093=CARTESIAN_POINT('',(-1.20190105810224,0.75,-0.335465908756113));
#11094=CARTESIAN_POINT('Origin',(-1.1682203282434,0.75,-0.379577794185951));
#11095=CARTESIAN_POINT('',(-1.22320001975977,0.75,-0.246749348660852));
#11096=CARTESIAN_POINT('Origin',(0.,0.75,0.));
#11097=CARTESIAN_POINT('',(-1.23958209161204,0.75,-0.143317017690053));
#11098=CARTESIAN_POINT('Origin',(-1.21321664662686,0.75,-0.192154639568406));
#11099=CARTESIAN_POINT('',(-1.24674050008925,0.75,-0.0523608139934482));
#11100=CARTESIAN_POINT('Origin',(0.,0.75,0.));
#11101=CARTESIAN_POINT('',(-1.24674050008925,0.75,0.0523608139934479));
#11102=CARTESIAN_POINT('Origin',(-1.22833954473516,0.75,-1.50428209172603E-16));
#11103=CARTESIAN_POINT('',(-1.23958209161204,0.75,0.143317017690053));
#11104=CARTESIAN_POINT('Origin',(0.,0.75,0.));
#11105=CARTESIAN_POINT('',(-1.22320001975977,0.75,0.246749348660851));
#11106=CARTESIAN_POINT('Origin',(-1.21321664662686,0.75,0.192154639568406));
#11107=CARTESIAN_POINT('',(-1.20190105810224,0.75,0.335465908756113));
#11108=CARTESIAN_POINT('Origin',(0.,0.75,0.));
#11109=CARTESIAN_POINT('',(-1.16954029537568,0.75,0.435062095450087));
#11110=CARTESIAN_POINT('Origin',(-1.1682203282434,0.75,0.379577794185951));
#11111=CARTESIAN_POINT('',(-1.13462523166105,0.75,0.519354515801077));
#11112=CARTESIAN_POINT('Origin',(0.,0.75,0.));
#11113=CARTESIAN_POINT('',(-1.08708260743774,0.75,0.612662169561028));
#11114=CARTESIAN_POINT('Origin',(-1.0944585482776,0.75,0.557654483764164));
#11115=CARTESIAN_POINT('',(-1.0394111664111,0.75,0.690454891028201));
#11116=CARTESIAN_POINT('Origin',(0.,0.75,0.));
#11117=CARTESIAN_POINT('',(-0.977857337884348,0.75,0.775176467748211));
#11118=CARTESIAN_POINT('Origin',(-0.993747566553533,0.75,0.721999869202979));
#11119=CARTESIAN_POINT('',(-0.918603348636233,0.75,0.844553975349804));
#11120=CARTESIAN_POINT('Origin',(0.,0.75,0.));
#11121=CARTESIAN_POINT('',(-0.844553975349804,0.75,0.918603348636233));
#11122=CARTESIAN_POINT('Origin',(-0.86856722168183,0.75,0.86856722168183));
#11123=CARTESIAN_POINT('',(-0.775176467748211,0.75,0.977857337884349));
#11124=CARTESIAN_POINT('Origin',(0.,0.75,0.));
#11125=CARTESIAN_POINT('',(-0.690454891028201,0.75,1.0394111664111));
#11126=CARTESIAN_POINT('Origin',(-0.721999869202979,0.75,0.993747566553533));
#11127=CARTESIAN_POINT('',(-0.612662169561029,0.75,1.08708260743774));
#11128=CARTESIAN_POINT('Origin',(0.,0.75,0.));
#11129=CARTESIAN_POINT('',(-0.519354515801077,0.75,1.13462523166105));
#11130=CARTESIAN_POINT('Origin',(-0.557654483764164,0.75,1.0944585482776));
#11131=CARTESIAN_POINT('',(-0.435062095450087,0.75,1.16954029537568));
#11132=CARTESIAN_POINT('Origin',(0.,0.75,0.));
#11133=CARTESIAN_POINT('',(-0.335465908756113,0.75,1.20190105810224));
#11134=CARTESIAN_POINT('Origin',(-0.379577794185951,0.75,1.1682203282434));
#11135=CARTESIAN_POINT('',(-0.246749348660852,0.75,1.22320001975977));
#11136=CARTESIAN_POINT('Origin',(0.,0.75,0.));
#11137=CARTESIAN_POINT('',(-0.143317017690053,0.75,1.23958209161204));
#11138=CARTESIAN_POINT('Origin',(-0.192154639568406,0.75,1.21321664662686));
#11139=CARTESIAN_POINT('',(-0.0523608139934483,0.75,1.24674050008925));
#11140=CARTESIAN_POINT('Origin',(0.,0.75,0.));
#11141=CARTESIAN_POINT('',(0.0523608139934478,0.75,1.24674050008925));
#11142=CARTESIAN_POINT('Origin',(-2.25642313758905E-16,0.75,1.22833954473516));
#11143=CARTESIAN_POINT('',(0.143317017690053,0.75,1.23958209161204));
#11144=CARTESIAN_POINT('Origin',(0.,0.75,0.));
#11145=CARTESIAN_POINT('',(0.246749348660851,0.75,1.22320001975977));
#11146=CARTESIAN_POINT('Origin',(0.192154639568406,0.75,1.21321664662686));
#11147=CARTESIAN_POINT('',(0.335465908756113,0.75,1.20190105810224));
#11148=CARTESIAN_POINT('Origin',(0.,0.75,0.));
#11149=CARTESIAN_POINT('',(0.435062095450087,0.75,1.16954029537568));
#11150=CARTESIAN_POINT('Origin',(0.379577794185951,0.75,1.1682203282434));
#11151=CARTESIAN_POINT('',(0.519354515801077,0.75,1.13462523166105));
#11152=CARTESIAN_POINT('Origin',(0.,0.75,0.));
#11153=CARTESIAN_POINT('',(0.612662169561028,0.75,1.08708260743774));
#11154=CARTESIAN_POINT('Origin',(0.557654483764164,0.75,1.0944585482776));
#11155=CARTESIAN_POINT('',(0.690454891028201,0.75,1.0394111664111));
#11156=CARTESIAN_POINT('Origin',(0.,0.75,0.));
#11157=CARTESIAN_POINT('',(0.775176467748211,0.75,0.977857337884349));
#11158=CARTESIAN_POINT('Origin',(0.721999869202979,0.75,0.993747566553533));
#11159=CARTESIAN_POINT('',(0.844553975349804,0.75,0.918603348636233));
#11160=CARTESIAN_POINT('Origin',(0.,0.75,0.));
#11161=CARTESIAN_POINT('',(0.918603348636233,0.75,0.844553975349804));
#11162=CARTESIAN_POINT('Origin',(0.86856722168183,0.75,0.86856722168183));
#11163=CARTESIAN_POINT('',(0.977857337884349,0.75,0.775176467748211));
#11164=CARTESIAN_POINT('Origin',(0.,0.75,0.));
#11165=CARTESIAN_POINT('',(1.0394111664111,0.75,0.690454891028201));
#11166=CARTESIAN_POINT('Origin',(0.993747566553533,0.75,0.72199986920298));
#11167=CARTESIAN_POINT('',(1.08708260743774,0.75,0.612662169561029));
#11168=CARTESIAN_POINT('Origin',(0.,0.75,0.));
#11169=CARTESIAN_POINT('',(1.13462523166105,0.75,0.519354515801077));
#11170=CARTESIAN_POINT('Origin',(1.0944585482776,0.75,0.557654483764164));
#11171=CARTESIAN_POINT('',(1.16954029537568,0.75,0.435062095450087));
#11172=CARTESIAN_POINT('Origin',(0.,0.75,0.));
#11173=CARTESIAN_POINT('',(1.20190105810224,0.75,0.335465908756113));
#11174=CARTESIAN_POINT('Origin',(1.1682203282434,0.75,0.379577794185952));
#11175=CARTESIAN_POINT('Origin',(0.,0.75,0.));
#11176=CARTESIAN_POINT('Origin',(0.,0.75,0.));
#11177=CARTESIAN_POINT('',(-1.4,0.75,1.71450551880629E-16));
#11178=CARTESIAN_POINT('Origin',(1.21321664662686,0.,0.192154639568406));
#11179=CARTESIAN_POINT('',(1.23958209161204,0.,0.14331701769005));
#11180=CARTESIAN_POINT('',(1.22320001975977,0.,0.246749348660855));
#11181=CARTESIAN_POINT('Origin',(0.,0.,0.));
#11182=CARTESIAN_POINT('',(1.20190105810224,0.,0.33546590875611));
#11183=CARTESIAN_POINT('Origin',(1.1682203282434,0.,0.379577794185952));
#11184=CARTESIAN_POINT('',(1.16954029537568,0.,0.43506209545009));
#11185=CARTESIAN_POINT('Origin',(0.,0.,0.));
#11186=CARTESIAN_POINT('',(1.13462523166105,0.,0.519354515801074));
#11187=CARTESIAN_POINT('Origin',(1.0944585482776,0.,0.557654483764164));
#11188=CARTESIAN_POINT('',(1.08708260743774,0.,0.612662169561031));
#11189=CARTESIAN_POINT('Origin',(0.,0.,0.));
#11190=CARTESIAN_POINT('',(1.03941116641111,0.,0.690454891028199));
#11191=CARTESIAN_POINT('Origin',(0.993747566553533,0.,0.72199986920298));
#11192=CARTESIAN_POINT('',(0.977857337884347,0.,0.775176467748214));
#11193=CARTESIAN_POINT('Origin',(0.,0.,0.));
#11194=CARTESIAN_POINT('',(0.918603348636235,0.,0.844553975349802));
#11195=CARTESIAN_POINT('Origin',(0.86856722168183,0.,0.86856722168183));
#11196=CARTESIAN_POINT('',(0.844553975349802,0.,0.918603348636235));
#11197=CARTESIAN_POINT('Origin',(0.,0.,0.));
#11198=CARTESIAN_POINT('',(0.775176467748213,0.,0.977857337884347));
#11199=CARTESIAN_POINT('Origin',(0.721999869202979,0.,0.993747566553533));
#11200=CARTESIAN_POINT('',(0.690454891028198,0.,1.03941116641111));
#11201=CARTESIAN_POINT('Origin',(0.,0.,0.));
#11202=CARTESIAN_POINT('',(0.612662169561031,0.,1.08708260743774));
#11203=CARTESIAN_POINT('Origin',(0.557654483764164,0.,1.0944585482776));
#11204=CARTESIAN_POINT('',(0.519354515801074,0.,1.13462523166105));
#11205=CARTESIAN_POINT('Origin',(0.,0.,0.));
#11206=CARTESIAN_POINT('',(0.43506209545009,0.,1.16954029537568));
#11207=CARTESIAN_POINT('Origin',(0.379577794185951,0.,1.1682203282434));
#11208=CARTESIAN_POINT('',(0.33546590875611,0.,1.20190105810224));
#11209=CARTESIAN_POINT('Origin',(0.,0.,0.));
#11210=CARTESIAN_POINT('',(0.246749348660854,0.,1.22320001975977));
#11211=CARTESIAN_POINT('Origin',(0.192154639568406,0.,1.21321664662686));
#11212=CARTESIAN_POINT('',(0.14331701769005,0.,1.23958209161204));
#11213=CARTESIAN_POINT('Origin',(0.,0.,0.));
#11214=CARTESIAN_POINT('',(0.0523608139934508,0.,1.24674050008925));
#11215=CARTESIAN_POINT('Origin',(-2.25642313758905E-16,0.,1.22833954473516));
#11216=CARTESIAN_POINT('',(-0.0523608139934513,0.,1.24674050008925));
#11217=CARTESIAN_POINT('Origin',(0.,0.,0.));
#11218=CARTESIAN_POINT('',(-0.14331701769005,0.,1.23958209161204));
#11219=CARTESIAN_POINT('Origin',(-0.192154639568406,0.,1.21321664662686));
#11220=CARTESIAN_POINT('',(-0.246749348660855,0.,1.22320001975977));
#11221=CARTESIAN_POINT('Origin',(0.,0.,0.));
#11222=CARTESIAN_POINT('',(-0.33546590875611,0.,1.20190105810224));
#11223=CARTESIAN_POINT('Origin',(-0.379577794185951,0.,1.1682203282434));
#11224=CARTESIAN_POINT('',(-0.43506209545009,0.,1.16954029537568));
#11225=CARTESIAN_POINT('Origin',(0.,0.,0.));
#11226=CARTESIAN_POINT('',(-0.519354515801074,0.,1.13462523166105));
#11227=CARTESIAN_POINT('Origin',(-0.557654483764164,0.,1.0944585482776));
#11228=CARTESIAN_POINT('',(-0.612662169561031,0.,1.08708260743774));
#11229=CARTESIAN_POINT('Origin',(0.,0.,0.));
#11230=CARTESIAN_POINT('',(-0.690454891028199,0.,1.03941116641111));
#11231=CARTESIAN_POINT('Origin',(-0.721999869202979,0.,0.993747566553533));
#11232=CARTESIAN_POINT('',(-0.775176467748213,0.,0.977857337884347));
#11233=CARTESIAN_POINT('Origin',(0.,0.,0.));
#11234=CARTESIAN_POINT('',(-0.844553975349802,0.,0.918603348636235));
#11235=CARTESIAN_POINT('Origin',(-0.86856722168183,0.,0.86856722168183));
#11236=CARTESIAN_POINT('',(-0.918603348636235,0.,0.844553975349802));
#11237=CARTESIAN_POINT('Origin',(0.,0.,0.));
#11238=CARTESIAN_POINT('',(-0.977857337884347,0.,0.775176467748213));
#11239=CARTESIAN_POINT('Origin',(-0.993747566553533,0.,0.721999869202979));
#11240=CARTESIAN_POINT('',(-1.03941116641111,0.,0.690454891028198));
#11241=CARTESIAN_POINT('Origin',(0.,0.,0.));
#11242=CARTESIAN_POINT('',(-1.08708260743774,0.,0.612662169561031));
#11243=CARTESIAN_POINT('Origin',(-1.0944585482776,0.,0.557654483764164));
#11244=CARTESIAN_POINT('',(-1.13462523166105,0.,0.519354515801074));
#11245=CARTESIAN_POINT('Origin',(0.,0.,0.));
#11246=CARTESIAN_POINT('',(-1.16954029537568,0.,0.43506209545009));
#11247=CARTESIAN_POINT('Origin',(-1.1682203282434,0.,0.379577794185951));
#11248=CARTESIAN_POINT('',(-1.20190105810224,0.,0.33546590875611));
#11249=CARTESIAN_POINT('Origin',(0.,0.,0.));
#11250=CARTESIAN_POINT('',(-1.22320001975977,0.,0.246749348660854));
#11251=CARTESIAN_POINT('Origin',(-1.21321664662686,0.,0.192154639568406));
#11252=CARTESIAN_POINT('',(-1.23958209161204,0.,0.14331701769005));
#11253=CARTESIAN_POINT('Origin',(0.,0.,0.));
#11254=CARTESIAN_POINT('',(-1.24674050008925,0.,0.0523608139934509));
#11255=CARTESIAN_POINT('Origin',(-1.22833954473516,0.,-1.50428209172603E-16));
#11256=CARTESIAN_POINT('',(-1.24674050008925,0.,-0.0523608139934512));
#11257=CARTESIAN_POINT('Origin',(0.,0.,0.));
#11258=CARTESIAN_POINT('',(-1.23958209161204,0.,-0.14331701769005));
#11259=CARTESIAN_POINT('Origin',(-1.21321664662686,0.,-0.192154639568406));
#11260=CARTESIAN_POINT('',(-1.22320001975977,0.,-0.246749348660855));
#11261=CARTESIAN_POINT('Origin',(0.,0.,0.));
#11262=CARTESIAN_POINT('',(-1.20190105810224,0.,-0.33546590875611));
#11263=CARTESIAN_POINT('Origin',(-1.1682203282434,0.,-0.379577794185951));
#11264=CARTESIAN_POINT('',(-1.16954029537568,0.,-0.43506209545009));
#11265=CARTESIAN_POINT('Origin',(0.,0.,0.));
#11266=CARTESIAN_POINT('',(-1.13462523166105,0.,-0.519354515801074));
#11267=CARTESIAN_POINT('Origin',(-1.0944585482776,0.,-0.557654483764164));
#11268=CARTESIAN_POINT('',(-1.08708260743774,0.,-0.612662169561031));
#11269=CARTESIAN_POINT('Origin',(0.,0.,0.));
#11270=CARTESIAN_POINT('',(-1.03941116641111,0.,-0.690454891028199));
#11271=CARTESIAN_POINT('Origin',(-0.993747566553533,0.,-0.721999869202979));
#11272=CARTESIAN_POINT('',(-0.977857337884347,0.,-0.775176467748213));
#11273=CARTESIAN_POINT('Origin',(0.,0.,0.));
#11274=CARTESIAN_POINT('',(-0.918603348636235,0.,-0.844553975349802));
#11275=CARTESIAN_POINT('Origin',(-0.86856722168183,0.,-0.86856722168183));
#11276=CARTESIAN_POINT('',(-0.844553975349802,0.,-0.918603348636235));
#11277=CARTESIAN_POINT('Origin',(0.,0.,0.));
#11278=CARTESIAN_POINT('',(-0.775176467748213,0.,-0.977857337884347));
#11279=CARTESIAN_POINT('Origin',(-0.721999869202979,0.,-0.993747566553533));
#11280=CARTESIAN_POINT('',(-0.690454891028198,0.,-1.03941116641111));
#11281=CARTESIAN_POINT('Origin',(0.,0.,0.));
#11282=CARTESIAN_POINT('',(-0.612662169561031,0.,-1.08708260743774));
#11283=CARTESIAN_POINT('Origin',(-0.557654483764164,0.,-1.0944585482776));
#11284=CARTESIAN_POINT('',(-0.519354515801074,0.,-1.13462523166105));
#11285=CARTESIAN_POINT('Origin',(0.,0.,0.));
#11286=CARTESIAN_POINT('',(-0.43506209545009,0.,-1.16954029537568));
#11287=CARTESIAN_POINT('Origin',(-0.379577794185951,0.,-1.1682203282434));
#11288=CARTESIAN_POINT('',(-0.33546590875611,0.,-1.20190105810224));
#11289=CARTESIAN_POINT('Origin',(0.,0.,0.));
#11290=CARTESIAN_POINT('',(-0.246749348660854,0.,-1.22320001975977));
#11291=CARTESIAN_POINT('Origin',(-0.192154639568406,0.,-1.21321664662686));
#11292=CARTESIAN_POINT('',(-0.14331701769005,0.,-1.23958209161204));
#11293=CARTESIAN_POINT('Origin',(0.,0.,0.));
#11294=CARTESIAN_POINT('',(-0.052360813993451,0.,-1.24674050008925));
#11295=CARTESIAN_POINT('Origin',(7.52141045863017E-17,0.,-1.22833954473516));
#11296=CARTESIAN_POINT('',(0.0523608139934511,0.,-1.24674050008925));
#11297=CARTESIAN_POINT('Origin',(0.,0.,0.));
#11298=CARTESIAN_POINT('',(0.14331701769005,0.,-1.23958209161204));
#11299=CARTESIAN_POINT('Origin',(0.192154639568406,0.,-1.21321664662686));
#11300=CARTESIAN_POINT('',(0.246749348660855,0.,-1.22320001975977));
#11301=CARTESIAN_POINT('Origin',(0.,0.,0.));
#11302=CARTESIAN_POINT('',(0.33546590875611,0.,-1.20190105810224));
#11303=CARTESIAN_POINT('Origin',(0.379577794185951,0.,-1.1682203282434));
#11304=CARTESIAN_POINT('',(0.43506209545009,0.,-1.16954029537568));
#11305=CARTESIAN_POINT('Origin',(0.,0.,0.));
#11306=CARTESIAN_POINT('',(0.519354515801074,0.,-1.13462523166105));
#11307=CARTESIAN_POINT('Origin',(0.557654483764164,0.,-1.0944585482776));
#11308=CARTESIAN_POINT('',(0.612662169561031,0.,-1.08708260743774));
#11309=CARTESIAN_POINT('Origin',(0.,0.,0.));
#11310=CARTESIAN_POINT('',(0.690454891028198,0.,-1.03941116641111));
#11311=CARTESIAN_POINT('Origin',(0.721999869202979,0.,-0.993747566553533));
#11312=CARTESIAN_POINT('',(0.775176467748213,0.,-0.977857337884347));
#11313=CARTESIAN_POINT('Origin',(0.,0.,0.));
#11314=CARTESIAN_POINT('',(0.844553975349802,0.,-0.918603348636235));
#11315=CARTESIAN_POINT('Origin',(0.86856722168183,0.,-0.86856722168183));
#11316=CARTESIAN_POINT('',(0.918603348636235,0.,-0.844553975349802));
#11317=CARTESIAN_POINT('Origin',(0.,0.,0.));
#11318=CARTESIAN_POINT('',(0.977857337884347,0.,-0.775176467748213));
#11319=CARTESIAN_POINT('Origin',(0.993747566553533,0.,-0.721999869202979));
#11320=CARTESIAN_POINT('',(1.03941116641111,0.,-0.690454891028198));
#11321=CARTESIAN_POINT('Origin',(0.,0.,0.));
#11322=CARTESIAN_POINT('',(1.08708260743774,0.,-0.612662169561031));
#11323=CARTESIAN_POINT('Origin',(1.0944585482776,0.,-0.557654483764164));
#11324=CARTESIAN_POINT('',(1.13462523166105,0.,-0.519354515801074));
#11325=CARTESIAN_POINT('Origin',(0.,0.,0.));
#11326=CARTESIAN_POINT('',(1.16954029537568,0.,-0.43506209545009));
#11327=CARTESIAN_POINT('Origin',(1.1682203282434,0.,-0.379577794185951));
#11328=CARTESIAN_POINT('',(1.20190105810224,0.,-0.33546590875611));
#11329=CARTESIAN_POINT('Origin',(0.,0.,0.));
#11330=CARTESIAN_POINT('',(1.22320001975977,0.,-0.246749348660855));
#11331=CARTESIAN_POINT('Origin',(1.21321664662686,0.,-0.192154639568406));
#11332=CARTESIAN_POINT('',(1.23958209161204,0.,-0.14331701769005));
#11333=CARTESIAN_POINT('Origin',(0.,0.,0.));
#11334=CARTESIAN_POINT('',(1.24674050008925,0.,0.052360813993451));
#11335=CARTESIAN_POINT('Origin',(1.22833954473516,0.,0.));
#11336=CARTESIAN_POINT('',(1.24674050008925,0.,-0.052360813993451));
#11337=CARTESIAN_POINT('Origin',(0.,0.,0.));
#11725=UNCERTAINTY_MEASURE_WITH_UNIT(LENGTH_MEASURE(0.001),#11765,
'DISTANCE_ACCURACY_VALUE',
'Maximum model space distance between geometric entities at asserted c
onnectivities');
#11732=UNCERTAINTY_MEASURE_WITH_UNIT(LENGTH_MEASURE(0.001),#11765,
'DISTANCE_ACCURACY_VALUE',
'Maximum model space distance between geometric entities at asserted c
onnectivities');
#11757=(
GEOMETRIC_REPRESENTATION_CONTEXT(3)
GLOBAL_UNCERTAINTY_ASSIGNED_CONTEXT((#11725))
GLOBAL_UNIT_ASSIGNED_CONTEXT((#11765,#11767,#11768))
REPRESENTATION_CONTEXT('','3D')
);
#11764=(
GEOMETRIC_REPRESENTATION_CONTEXT(3)
GLOBAL_UNCERTAINTY_ASSIGNED_CONTEXT((#11732))
GLOBAL_UNIT_ASSIGNED_CONTEXT((#11765,#11767,#11768))
REPRESENTATION_CONTEXT('','3D')
);
#11765=(
LENGTH_UNIT()
NAMED_UNIT(*)
SI_UNIT(.CENTI.,.METRE.)
);
#11767=(
NAMED_UNIT(*)
PLANE_ANGLE_UNIT()
SI_UNIT($,.RADIAN.)
);
#11768=(
NAMED_UNIT(*)
SI_UNIT($,.STERADIAN.)
SOLID_ANGLE_UNIT()
);
#11793=SHAPE_DEFINITION_REPRESENTATION(#11826,#11902);
#11826=PRODUCT_DEFINITION_SHAPE('',$,#11934);
#11902=SHAPE_REPRESENTATION('',(#6807),#11757);
#11909=PRODUCT_DEFINITION_CONTEXT('part definition',#12004,'design');
#11934=PRODUCT_DEFINITION(
'Timing Pulley - 2 mm Pitch, 40 Teeth, 12 mm Bore',
'Timing Pulley - 2 mm Pitch, 40 Teeth, 12 mm Bore',#11965,#11909);
#11965=PRODUCT_DEFINITION_FORMATION('',$,#12030);
#12004=APPLICATION_CONTEXT(
'Core Data for Automotive Mechanical Design Process');
#12005=PRODUCT_CONTEXT('part definition',#12004,'mechanical');
#12030=PRODUCT('Timing Pulley - 2 mm Pitch, 40 Teeth, 12 mm Bore',
'Timing Pulley - 2 mm Pitch, 40 Teeth, 12 mm Bore',
'Timing Pulley - 2 mm Pitch, 40 Teeth, 12 mm Bore',(#12005));
#12086=COLOUR_RGB('Sky Blue',0.24,0.69,0.87);
#12087=FILL_AREA_STYLE_COLOUR('',#12086);
#12088=FILL_AREA_STYLE('',(#12087));
#12089=SURFACE_STYLE_FILL_AREA(#12088);
#12090=SURFACE_SIDE_STYLE('',(#12089));
#12091=SURFACE_STYLE_USAGE(.BOTH.,#12090);
#12092=PRESENTATION_STYLE_ASSIGNMENT((#12091));
ENDSEC;
END-ISO-10303-21;
